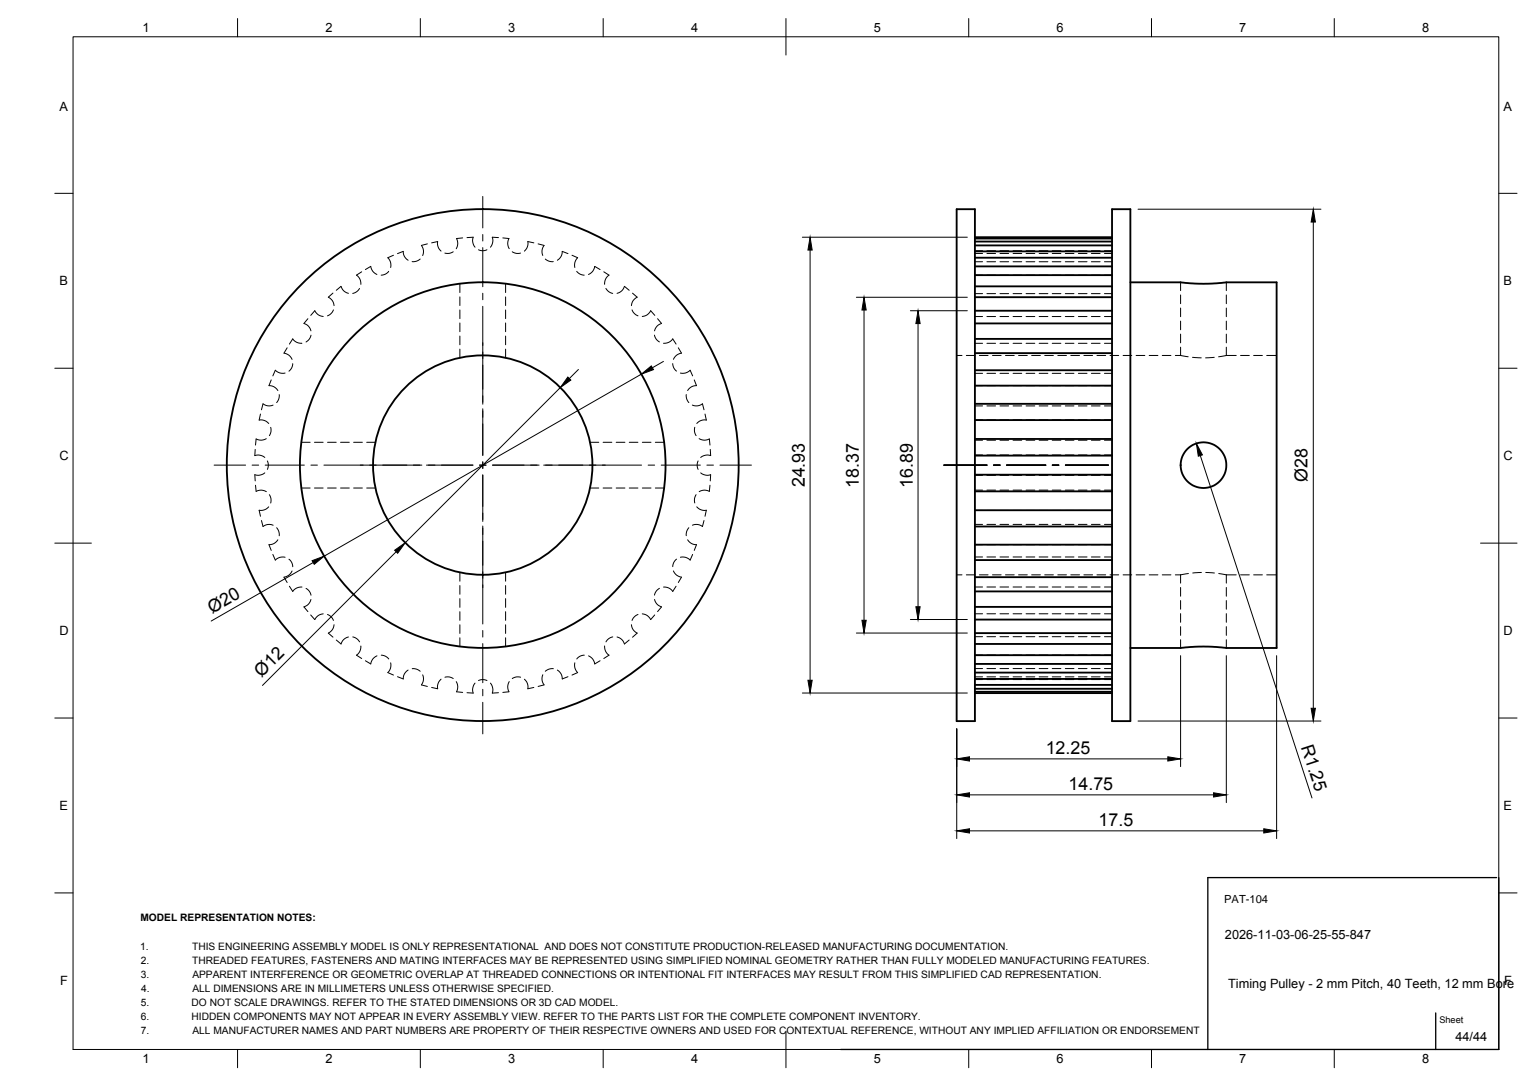
ISO-10303-21;
HEADER;
/* Generated by software containing ST-Developer
 * from STEP Tools, Inc. (www.steptools.com) 
 */

FILE_DESCRIPTION(
/* description */ ('Timing belt drive module 2 mm Pitch Timing 20T-40T'),

/* implementation_level */ '2;1');

FILE_NAME(
/* name */ 'Timing Pulley - 2 mm Pitch, 40 Teeth, 12 mm Bore.step',
/* time_stamp */ '2026-10-28T03:25:12-07:00',
/* author */ (''),
/* organization */ (''),
/* preprocessor_version */ 'ST-DEVELOPER v20.2',
/* originating_system */ 'Autodesk Translation Framework v15.17.0.0',
/* authorisation */ '');

FILE_SCHEMA (('AUTOMOTIVE_DESIGN { 1 0 10303 214 3 1 1 }'));
ENDSEC;

DATA;
#10=MECHANICAL_DESIGN_GEOMETRIC_PRESENTATION_REPRESENTATION('',(#580),#17830);
#363=B_SPLINE_CURVE_WITH_KNOTS('',3,(#16760,#16761,#16762,#16763,#16764,
#16765,#16766,#16767,#16768,#16769),.UNSPECIFIED.,.F.,.F.,(4,2,2,2,4),(0.565665723963061,
0.61280433739166,0.659942950820258,0.70708195805217,0.754220965284082),
 .UNSPECIFIED.);
#364=B_SPLINE_CURVE_WITH_KNOTS('',3,(#16771,#16772,#16773,#16774,#16775,
#16776,#16777,#16778,#16779,#16780,#16781,#16782,#16783,#16784,#16785,#16786,
#16787,#16788),.UNSPECIFIED.,.F.,.F.,(4,2,2,2,2,2,2,2,4),(0.18855524132102,
0.235693854749619,0.282832468178217,0.329971475410129,0.377110482642041,
0.424249489873953,0.471388497105864,0.518527110534463,0.565665723963061),
 .UNSPECIFIED.);
#365=B_SPLINE_CURVE_WITH_KNOTS('',3,(#16789,#16790,#16791,#16792,#16793,
#16794,#16795,#16796,#16797,#16798),.UNSPECIFIED.,.F.,.F.,(4,2,2,2,4),(0.754220965284082,
0.801359972515993,0.848498979747905,0.895637593176504,0.942776206605102),
 .UNSPECIFIED.);
#366=B_SPLINE_CURVE_WITH_KNOTS('',3,(#16802,#16803,#16804,#16805,#16806,
#16807,#16808,#16809,#16810,#16811),.UNSPECIFIED.,.F.,.F.,(4,2,2,2,4),(0.188940047579712,
0.236173496177583,0.283406944775455,0.330643519967439,0.377880095159423),
 .UNSPECIFIED.);
#367=B_SPLINE_CURVE_WITH_KNOTS('',3,(#16813,#16814,#16815,#16816,#16817,
#16818,#16819,#16820,#16821,#16822),.UNSPECIFIED.,.F.,.F.,(4,2,2,2,4),(0.,
0.0472365751919841,0.0944731503839682,0.14170659898184,0.188940047579712),
 .UNSPECIFIED.);
#368=B_SPLINE_CURVE_WITH_KNOTS('',3,(#16824,#16825,#16826,#16827,#16828,
#16829,#16830,#16831,#16832,#16833),.UNSPECIFIED.,.F.,.F.,(4,2,2,2,4),(0.566820142739135,
0.614053591337007,0.661287039934879,0.708523615126863,0.755760190318847),
 .UNSPECIFIED.);
#369=B_SPLINE_CURVE_WITH_KNOTS('',3,(#16834,#16835,#16836,#16837,#16838,
#16839,#16840,#16841,#16842,#16843),.UNSPECIFIED.,.F.,.F.,(4,2,2,2,4),(0.377880095159423,
0.425116670351408,0.472353245543392,0.519586694141263,0.566820142739135),
 .UNSPECIFIED.);
#370=B_SPLINE_CURVE_WITH_KNOTS('',3,(#16847,#16848,#16849,#16850,#16851,
#16852,#16853,#16854,#16855,#16856,#16857,#16858,#16859,#16860,#16861,#16862,
#16863,#16864),.UNSPECIFIED.,.F.,.F.,(4,2,2,2,2,2,2,2,4),(0.,0.0472365751919841,
0.0944731503839683,0.14170659898184,0.188940047579712,0.236173496177583,
0.283406944775455,0.330643519967439,0.377880095159423),.UNSPECIFIED.);
#371=B_SPLINE_CURVE_WITH_KNOTS('',3,(#16865,#16866,#16867,#16868,#16869,
#16870,#16871,#16872,#16873,#16874,#16875,#16876,#16877,#16878,#16879,#16880,
#16881,#16882),.UNSPECIFIED.,.F.,.F.,(4,2,2,2,2,2,2,2,4),(0.377880095159423,
0.425116670351408,0.472353245543392,0.519586694141263,0.566820142739135,
0.614053591337007,0.661287039934879,0.708523615126863,0.755760190318847),
 .UNSPECIFIED.);
#372=B_SPLINE_CURVE_WITH_KNOTS('',3,(#16886,#16887,#16888,#16889,#16890,
#16891,#16892,#16893,#16894,#16895),.UNSPECIFIED.,.F.,.F.,(4,2,2,2,4),(0.565665723963061,
0.61280433739166,0.659942950820258,0.70708195805217,0.754220965284082),
 .UNSPECIFIED.);
#373=B_SPLINE_CURVE_WITH_KNOTS('',3,(#16897,#16898,#16899,#16900,#16901,
#16902,#16903,#16904,#16905,#16906,#16907,#16908,#16909,#16910,#16911,#16912,
#16913,#16914),.UNSPECIFIED.,.F.,.F.,(4,2,2,2,2,2,2,2,4),(0.18855524132102,
0.235693854749619,0.282832468178217,0.329971475410129,0.377110482642041,
0.424249489873953,0.471388497105864,0.518527110534463,0.565665723963061),
 .UNSPECIFIED.);
#374=B_SPLINE_CURVE_WITH_KNOTS('',3,(#16915,#16916,#16917,#16918,#16919,
#16920,#16921,#16922,#16923,#16924),.UNSPECIFIED.,.F.,.F.,(4,2,2,2,4),(0.754220965284082,
0.801359972515993,0.848498979747905,0.895637593176504,0.942776206605102),
 .UNSPECIFIED.);
#375=B_SPLINE_CURVE_WITH_KNOTS('',3,(#16934,#16935,#16936,#16937,#16938,
#16939,#16940,#16941,#16942,#16943,#16944,#16945,#16946,#16947,#16948,#16949,
#16950,#16951),.UNSPECIFIED.,.F.,.F.,(4,2,2,2,2,2,2,2,4),(0.18855524132102,
0.235693854749619,0.282832468178217,0.329971475410129,0.377110482642041,
0.424249489873953,0.471388497105864,0.518527110534463,0.565665723963061),
 .UNSPECIFIED.);
#376=B_SPLINE_CURVE_WITH_KNOTS('',3,(#16953,#16954,#16955,#16956,#16957,
#16958,#16959,#16960,#16961,#16962),.UNSPECIFIED.,.F.,.F.,(4,2,2,2,4),(0.565665723963061,
0.61280433739166,0.659942950820258,0.70708195805217,0.754220965284082),
 .UNSPECIFIED.);
#377=B_SPLINE_CURVE_WITH_KNOTS('',3,(#16963,#16964,#16965,#16966,#16967,
#16968,#16969,#16970,#16971,#16972),.UNSPECIFIED.,.F.,.F.,(4,2,2,2,4),(0.754220965284082,
0.801359972515993,0.848498979747905,0.895637593176504,0.942776206605102),
 .UNSPECIFIED.);
#378=B_SPLINE_CURVE_WITH_KNOTS('',3,(#16975,#16976,#16977,#16978,#16979,
#16980,#16981,#16982,#16983,#16984,#16985,#16986,#16987,#16988,#16989,#16990,
#16991,#16992),.UNSPECIFIED.,.F.,.F.,(4,2,2,2,2,2,2,2,4),(0.18855524132102,
0.235693854749619,0.282832468178217,0.329971475410129,0.377110482642041,
0.424249489873953,0.471388497105864,0.518527110534463,0.565665723963061),
 .UNSPECIFIED.);
#379=B_SPLINE_CURVE_WITH_KNOTS('',3,(#16994,#16995,#16996,#16997,#16998,
#16999,#17000,#17001,#17002,#17003),.UNSPECIFIED.,.F.,.F.,(4,2,2,2,4),(0.565665723963061,
0.61280433739166,0.659942950820258,0.70708195805217,0.754220965284082),
 .UNSPECIFIED.);
#380=B_SPLINE_CURVE_WITH_KNOTS('',3,(#17004,#17005,#17006,#17007,#17008,
#17009,#17010,#17011,#17012,#17013),.UNSPECIFIED.,.F.,.F.,(4,2,2,2,4),(0.754220965284082,
0.801359972515993,0.848498979747905,0.895637593176504,0.942776206605102),
 .UNSPECIFIED.);
#381=B_SPLINE_CURVE_WITH_KNOTS('',3,(#17018,#17019,#17020,#17021,#17022,
#17023,#17024,#17025,#17026,#17027,#17028,#17029,#17030,#17031,#17032,#17033,
#17034,#17035),.UNSPECIFIED.,.F.,.F.,(4,2,2,2,2,2,2,2,4),(0.,0.0472365751919841,
0.0944731503839683,0.14170659898184,0.188940047579712,0.236173496177583,
0.283406944775455,0.330643519967439,0.377880095159424),.UNSPECIFIED.);
#382=B_SPLINE_CURVE_WITH_KNOTS('',3,(#17036,#17037,#17038,#17039,#17040,
#17041,#17042,#17043,#17044,#17045,#17046,#17047,#17048,#17049,#17050,#17051,
#17052,#17053),.UNSPECIFIED.,.F.,.F.,(4,2,2,2,2,2,2,2,4),(0.377880095159424,
0.425116670351408,0.472353245543392,0.519586694141263,0.566820142739135,
0.614053591337007,0.661287039934879,0.708523615126863,0.755760190318847),
 .UNSPECIFIED.);
#383=B_SPLINE_CURVE_WITH_KNOTS('',3,(#17057,#17058,#17059,#17060,#17061,
#17062,#17063,#17064,#17065,#17066,#17067,#17068,#17069,#17070,#17071,#17072,
#17073,#17074),.UNSPECIFIED.,.F.,.F.,(4,2,2,2,2,2,2,2,4),(0.,0.0472365751919841,
0.0944731503839683,0.14170659898184,0.188940047579712,0.236173496177583,
0.283406944775455,0.330643519967439,0.377880095159423),.UNSPECIFIED.);
#384=B_SPLINE_CURVE_WITH_KNOTS('',3,(#17075,#17076,#17077,#17078,#17079,
#17080,#17081,#17082,#17083,#17084,#17085,#17086,#17087,#17088,#17089,#17090,
#17091,#17092),.UNSPECIFIED.,.F.,.F.,(4,2,2,2,2,2,2,2,4),(0.377880095159423,
0.425116670351408,0.472353245543392,0.519586694141263,0.566820142739135,
0.614053591337007,0.661287039934879,0.708523615126863,0.755760190318847),
 .UNSPECIFIED.);
#479=SHAPE_REPRESENTATION_RELATIONSHIP('SRR','None',#18053,#522);
#522=ADVANCED_BREP_SHAPE_REPRESENTATION('',(#636),#17828);
#580=STYLED_ITEM('',(#18310),#636);
#636=MANIFOLD_SOLID_BREP('Body1',#9039);
#761=FACE_BOUND('',#2021,.T.);
#762=FACE_BOUND('',#2022,.T.);
#763=FACE_BOUND('',#2023,.T.);
#764=FACE_BOUND('',#2027,.T.);
#765=FACE_BOUND('',#2028,.T.);
#766=FACE_BOUND('',#2029,.T.);
#767=FACE_BOUND('',#2031,.T.);
#768=FACE_BOUND('',#2033,.T.);
#769=FACE_BOUND('',#2036,.T.);
#770=FACE_BOUND('',#2038,.T.);
#771=FACE_BOUND('',#2041,.T.);
#946=PLANE('',#10469);
#947=PLANE('',#10470);
#948=PLANE('',#10554);
#949=PLANE('',#10555);
#950=PLANE('',#10639);
#1373=FACE_OUTER_BOUND('',#2018,.T.);
#1374=FACE_OUTER_BOUND('',#2019,.T.);
#1375=FACE_OUTER_BOUND('',#2020,.T.);
#1376=FACE_OUTER_BOUND('',#2024,.T.);
#1377=FACE_OUTER_BOUND('',#2025,.T.);
#1378=FACE_OUTER_BOUND('',#2026,.T.);
#1379=FACE_OUTER_BOUND('',#2030,.T.);
#1380=FACE_OUTER_BOUND('',#2032,.T.);
#1381=FACE_OUTER_BOUND('',#2034,.T.);
#1382=FACE_OUTER_BOUND('',#2035,.T.);
#1383=FACE_OUTER_BOUND('',#2037,.T.);
#1384=FACE_OUTER_BOUND('',#2039,.T.);
#1385=FACE_OUTER_BOUND('',#2040,.T.);
#1386=FACE_OUTER_BOUND('',#2042,.T.);
#1387=FACE_OUTER_BOUND('',#2043,.T.);
#1388=FACE_OUTER_BOUND('',#2044,.T.);
#1389=FACE_OUTER_BOUND('',#2045,.T.);
#1390=FACE_OUTER_BOUND('',#2046,.T.);
#1391=FACE_OUTER_BOUND('',#2047,.T.);
#1392=FACE_OUTER_BOUND('',#2048,.T.);
#1393=FACE_OUTER_BOUND('',#2049,.T.);
#1394=FACE_OUTER_BOUND('',#2050,.T.);
#1395=FACE_OUTER_BOUND('',#2051,.T.);
#1396=FACE_OUTER_BOUND('',#2052,.T.);
#1397=FACE_OUTER_BOUND('',#2053,.T.);
#1398=FACE_OUTER_BOUND('',#2054,.T.);
#1399=FACE_OUTER_BOUND('',#2055,.T.);
#1400=FACE_OUTER_BOUND('',#2056,.T.);
#1401=FACE_OUTER_BOUND('',#2057,.T.);
#1402=FACE_OUTER_BOUND('',#2058,.T.);
#1403=FACE_OUTER_BOUND('',#2059,.T.);
#1404=FACE_OUTER_BOUND('',#2060,.T.);
#1405=FACE_OUTER_BOUND('',#2061,.T.);
#1406=FACE_OUTER_BOUND('',#2062,.T.);
#1407=FACE_OUTER_BOUND('',#2063,.T.);
#1408=FACE_OUTER_BOUND('',#2064,.T.);
#1409=FACE_OUTER_BOUND('',#2065,.T.);
#1410=FACE_OUTER_BOUND('',#2066,.T.);
#1411=FACE_OUTER_BOUND('',#2067,.T.);
#1412=FACE_OUTER_BOUND('',#2068,.T.);
#1413=FACE_OUTER_BOUND('',#2069,.T.);
#1414=FACE_OUTER_BOUND('',#2070,.T.);
#1415=FACE_OUTER_BOUND('',#2071,.T.);
#1416=FACE_OUTER_BOUND('',#2072,.T.);
#1417=FACE_OUTER_BOUND('',#2073,.T.);
#1418=FACE_OUTER_BOUND('',#2074,.T.);
#1419=FACE_OUTER_BOUND('',#2075,.T.);
#1420=FACE_OUTER_BOUND('',#2076,.T.);
#1421=FACE_OUTER_BOUND('',#2077,.T.);
#1422=FACE_OUTER_BOUND('',#2078,.T.);
#1423=FACE_OUTER_BOUND('',#2079,.T.);
#1424=FACE_OUTER_BOUND('',#2080,.T.);
#1425=FACE_OUTER_BOUND('',#2081,.T.);
#1426=FACE_OUTER_BOUND('',#2082,.T.);
#1427=FACE_OUTER_BOUND('',#2083,.T.);
#1428=FACE_OUTER_BOUND('',#2084,.T.);
#1429=FACE_OUTER_BOUND('',#2085,.T.);
#1430=FACE_OUTER_BOUND('',#2086,.T.);
#1431=FACE_OUTER_BOUND('',#2087,.T.);
#1432=FACE_OUTER_BOUND('',#2088,.T.);
#1433=FACE_OUTER_BOUND('',#2089,.T.);
#1434=FACE_OUTER_BOUND('',#2090,.T.);
#1435=FACE_OUTER_BOUND('',#2091,.T.);
#1436=FACE_OUTER_BOUND('',#2092,.T.);
#1437=FACE_OUTER_BOUND('',#2093,.T.);
#1438=FACE_OUTER_BOUND('',#2094,.T.);
#1439=FACE_OUTER_BOUND('',#2095,.T.);
#1440=FACE_OUTER_BOUND('',#2096,.T.);
#1441=FACE_OUTER_BOUND('',#2097,.T.);
#1442=FACE_OUTER_BOUND('',#2098,.T.);
#1443=FACE_OUTER_BOUND('',#2099,.T.);
#1444=FACE_OUTER_BOUND('',#2100,.T.);
#1445=FACE_OUTER_BOUND('',#2101,.T.);
#1446=FACE_OUTER_BOUND('',#2102,.T.);
#1447=FACE_OUTER_BOUND('',#2103,.T.);
#1448=FACE_OUTER_BOUND('',#2104,.T.);
#1449=FACE_OUTER_BOUND('',#2105,.T.);
#1450=FACE_OUTER_BOUND('',#2106,.T.);
#1451=FACE_OUTER_BOUND('',#2107,.T.);
#1452=FACE_OUTER_BOUND('',#2108,.T.);
#1453=FACE_OUTER_BOUND('',#2109,.T.);
#1454=FACE_OUTER_BOUND('',#2110,.T.);
#1455=FACE_OUTER_BOUND('',#2111,.T.);
#1456=FACE_OUTER_BOUND('',#2112,.T.);
#1457=FACE_OUTER_BOUND('',#2113,.T.);
#1458=FACE_OUTER_BOUND('',#2114,.T.);
#1459=FACE_OUTER_BOUND('',#2115,.T.);
#1460=FACE_OUTER_BOUND('',#2116,.T.);
#1461=FACE_OUTER_BOUND('',#2117,.T.);
#1462=FACE_OUTER_BOUND('',#2118,.T.);
#1463=FACE_OUTER_BOUND('',#2119,.T.);
#1464=FACE_OUTER_BOUND('',#2120,.T.);
#1465=FACE_OUTER_BOUND('',#2121,.T.);
#2018=EDGE_LOOP('',(#7557,#7558,#7559,#7560,#7561,#7562,#7563,#7564,#7565));
#2019=EDGE_LOOP('',(#7566,#7567,#7568,#7569,#7570,#7571,#7572));
#2020=EDGE_LOOP('',(#7573,#7574,#7575,#7576,#7577,#7578,#7579,#7580,#7581));
#2021=EDGE_LOOP('',(#7582,#7583,#7584));
#2022=EDGE_LOOP('',(#7585,#7586,#7587));
#2023=EDGE_LOOP('',(#7588,#7589,#7590));
#2024=EDGE_LOOP('',(#7591,#7592,#7593,#7594,#7595,#7596,#7597));
#2025=EDGE_LOOP('',(#7598,#7599,#7600,#7601,#7602,#7603,#7604));
#2026=EDGE_LOOP('',(#7605,#7606,#7607,#7608,#7609,#7610,#7611,#7612,#7613,
#7614));
#2027=EDGE_LOOP('',(#7615,#7616));
#2028=EDGE_LOOP('',(#7617,#7618));
#2029=EDGE_LOOP('',(#7619,#7620));
#2030=EDGE_LOOP('',(#7621));
#2031=EDGE_LOOP('',(#7622));
#2032=EDGE_LOOP('',(#7623));
#2033=EDGE_LOOP('',(#7624,#7625,#7626,#7627,#7628,#7629,#7630,#7631,#7632,
#7633,#7634,#7635,#7636,#7637,#7638,#7639,#7640,#7641,#7642,#7643,#7644,
#7645,#7646,#7647,#7648,#7649,#7650,#7651,#7652,#7653,#7654,#7655,#7656,
#7657,#7658,#7659,#7660,#7661,#7662,#7663,#7664,#7665,#7666,#7667,#7668,
#7669,#7670,#7671,#7672,#7673,#7674,#7675,#7676,#7677,#7678,#7679,#7680,
#7681,#7682,#7683,#7684,#7685,#7686,#7687,#7688,#7689,#7690,#7691,#7692,
#7693,#7694,#7695,#7696,#7697,#7698,#7699,#7700,#7701,#7702,#7703));
#2034=EDGE_LOOP('',(#7704,#7705,#7706,#7707));
#2035=EDGE_LOOP('',(#7708));
#2036=EDGE_LOOP('',(#7709));
#2037=EDGE_LOOP('',(#7710));
#2038=EDGE_LOOP('',(#7711,#7712,#7713,#7714,#7715,#7716,#7717,#7718,#7719,
#7720,#7721,#7722,#7723,#7724,#7725,#7726,#7727,#7728,#7729,#7730,#7731,
#7732,#7733,#7734,#7735,#7736,#7737,#7738,#7739,#7740,#7741,#7742,#7743,
#7744,#7745,#7746,#7747,#7748,#7749,#7750,#7751,#7752,#7753,#7754,#7755,
#7756,#7757,#7758,#7759,#7760,#7761,#7762,#7763,#7764,#7765,#7766,#7767,
#7768,#7769,#7770,#7771,#7772,#7773,#7774,#7775,#7776,#7777,#7778,#7779,
#7780,#7781,#7782,#7783,#7784,#7785,#7786,#7787,#7788,#7789,#7790));
#2039=EDGE_LOOP('',(#7791,#7792,#7793,#7794));
#2040=EDGE_LOOP('',(#7795));
#2041=EDGE_LOOP('',(#7796));
#2042=EDGE_LOOP('',(#7797,#7798,#7799,#7800));
#2043=EDGE_LOOP('',(#7801,#7802,#7803,#7804));
#2044=EDGE_LOOP('',(#7805,#7806,#7807,#7808));
#2045=EDGE_LOOP('',(#7809,#7810,#7811,#7812));
#2046=EDGE_LOOP('',(#7813,#7814,#7815,#7816));
#2047=EDGE_LOOP('',(#7817,#7818,#7819,#7820));
#2048=EDGE_LOOP('',(#7821,#7822,#7823,#7824));
#2049=EDGE_LOOP('',(#7825,#7826,#7827,#7828));
#2050=EDGE_LOOP('',(#7829,#7830,#7831,#7832));
#2051=EDGE_LOOP('',(#7833,#7834,#7835,#7836));
#2052=EDGE_LOOP('',(#7837,#7838,#7839,#7840));
#2053=EDGE_LOOP('',(#7841,#7842,#7843,#7844));
#2054=EDGE_LOOP('',(#7845,#7846,#7847,#7848));
#2055=EDGE_LOOP('',(#7849,#7850,#7851,#7852));
#2056=EDGE_LOOP('',(#7853,#7854,#7855,#7856));
#2057=EDGE_LOOP('',(#7857,#7858,#7859,#7860));
#2058=EDGE_LOOP('',(#7861,#7862,#7863,#7864));
#2059=EDGE_LOOP('',(#7865,#7866,#7867,#7868));
#2060=EDGE_LOOP('',(#7869,#7870,#7871,#7872));
#2061=EDGE_LOOP('',(#7873,#7874,#7875,#7876));
#2062=EDGE_LOOP('',(#7877,#7878,#7879,#7880));
#2063=EDGE_LOOP('',(#7881,#7882,#7883,#7884));
#2064=EDGE_LOOP('',(#7885,#7886,#7887,#7888));
#2065=EDGE_LOOP('',(#7889,#7890,#7891,#7892));
#2066=EDGE_LOOP('',(#7893,#7894,#7895,#7896));
#2067=EDGE_LOOP('',(#7897,#7898,#7899,#7900));
#2068=EDGE_LOOP('',(#7901,#7902,#7903,#7904));
#2069=EDGE_LOOP('',(#7905,#7906,#7907,#7908));
#2070=EDGE_LOOP('',(#7909,#7910,#7911,#7912));
#2071=EDGE_LOOP('',(#7913,#7914,#7915,#7916));
#2072=EDGE_LOOP('',(#7917,#7918,#7919,#7920));
#2073=EDGE_LOOP('',(#7921,#7922,#7923,#7924));
#2074=EDGE_LOOP('',(#7925,#7926,#7927,#7928));
#2075=EDGE_LOOP('',(#7929,#7930,#7931,#7932));
#2076=EDGE_LOOP('',(#7933,#7934,#7935,#7936));
#2077=EDGE_LOOP('',(#7937,#7938,#7939,#7940));
#2078=EDGE_LOOP('',(#7941,#7942,#7943,#7944));
#2079=EDGE_LOOP('',(#7945,#7946,#7947,#7948));
#2080=EDGE_LOOP('',(#7949,#7950,#7951,#7952));
#2081=EDGE_LOOP('',(#7953,#7954,#7955,#7956));
#2082=EDGE_LOOP('',(#7957,#7958,#7959,#7960));
#2083=EDGE_LOOP('',(#7961,#7962,#7963,#7964));
#2084=EDGE_LOOP('',(#7965,#7966,#7967,#7968));
#2085=EDGE_LOOP('',(#7969,#7970,#7971,#7972));
#2086=EDGE_LOOP('',(#7973,#7974,#7975,#7976));
#2087=EDGE_LOOP('',(#7977,#7978,#7979,#7980));
#2088=EDGE_LOOP('',(#7981,#7982,#7983,#7984));
#2089=EDGE_LOOP('',(#7985,#7986,#7987,#7988));
#2090=EDGE_LOOP('',(#7989,#7990,#7991,#7992));
#2091=EDGE_LOOP('',(#7993,#7994,#7995,#7996));
#2092=EDGE_LOOP('',(#7997,#7998,#7999,#8000));
#2093=EDGE_LOOP('',(#8001,#8002,#8003,#8004));
#2094=EDGE_LOOP('',(#8005,#8006,#8007,#8008));
#2095=EDGE_LOOP('',(#8009,#8010,#8011,#8012));
#2096=EDGE_LOOP('',(#8013,#8014,#8015,#8016));
#2097=EDGE_LOOP('',(#8017,#8018,#8019,#8020));
#2098=EDGE_LOOP('',(#8021,#8022,#8023,#8024));
#2099=EDGE_LOOP('',(#8025,#8026,#8027,#8028));
#2100=EDGE_LOOP('',(#8029,#8030,#8031,#8032));
#2101=EDGE_LOOP('',(#8033,#8034,#8035,#8036));
#2102=EDGE_LOOP('',(#8037,#8038,#8039,#8040));
#2103=EDGE_LOOP('',(#8041,#8042,#8043,#8044));
#2104=EDGE_LOOP('',(#8045,#8046,#8047,#8048));
#2105=EDGE_LOOP('',(#8049,#8050,#8051,#8052));
#2106=EDGE_LOOP('',(#8053,#8054,#8055,#8056));
#2107=EDGE_LOOP('',(#8057,#8058,#8059,#8060));
#2108=EDGE_LOOP('',(#8061,#8062,#8063,#8064));
#2109=EDGE_LOOP('',(#8065,#8066,#8067,#8068));
#2110=EDGE_LOOP('',(#8069,#8070,#8071,#8072));
#2111=EDGE_LOOP('',(#8073,#8074,#8075,#8076));
#2112=EDGE_LOOP('',(#8077,#8078,#8079,#8080));
#2113=EDGE_LOOP('',(#8081,#8082,#8083,#8084));
#2114=EDGE_LOOP('',(#8085,#8086,#8087,#8088));
#2115=EDGE_LOOP('',(#8089,#8090,#8091,#8092));
#2116=EDGE_LOOP('',(#8093,#8094,#8095,#8096));
#2117=EDGE_LOOP('',(#8097,#8098,#8099,#8100));
#2118=EDGE_LOOP('',(#8101,#8102,#8103,#8104));
#2119=EDGE_LOOP('',(#8105,#8106,#8107,#8108));
#2120=EDGE_LOOP('',(#8109,#8110,#8111,#8112));
#2121=EDGE_LOOP('',(#8113,#8114,#8115,#8116));
#2614=CIRCLE('',#10462,1.);
#2615=CIRCLE('',#10463,1.);
#2616=CIRCLE('',#10467,0.6);
#2617=CIRCLE('',#10468,0.6);
#2618=CIRCLE('',#10471,1.4);
#2619=CIRCLE('',#10472,0.0555000000000001);
#2620=CIRCLE('',#10473,1.24783954473516);
#2621=CIRCLE('',#10474,0.0555000000000001);
#2622=CIRCLE('',#10475,1.24783954473516);
#2623=CIRCLE('',#10476,0.0555000000000001);
#2624=CIRCLE('',#10477,1.24783954473516);
#2625=CIRCLE('',#10478,0.0555000000000001);
#2626=CIRCLE('',#10479,1.24783954473516);
#2627=CIRCLE('',#10480,0.0555000000000001);
#2628=CIRCLE('',#10481,1.24783954473516);
#2629=CIRCLE('',#10482,0.0555000000000001);
#2630=CIRCLE('',#10483,1.24783954473516);
#2631=CIRCLE('',#10484,0.0555000000000001);
#2632=CIRCLE('',#10485,1.24783954473516);
#2633=CIRCLE('',#10486,0.0555000000000001);
#2634=CIRCLE('',#10487,1.24783954473516);
#2635=CIRCLE('',#10488,0.0555000000000001);
#2636=CIRCLE('',#10489,1.24783954473516);
#2637=CIRCLE('',#10490,0.0555000000000001);
#2638=CIRCLE('',#10491,1.24783954473516);
#2639=CIRCLE('',#10492,0.0555000000000001);
#2640=CIRCLE('',#10493,1.24783954473516);
#2641=CIRCLE('',#10494,0.0555000000000001);
#2642=CIRCLE('',#10495,1.24783954473516);
#2643=CIRCLE('',#10496,0.0555000000000001);
#2644=CIRCLE('',#10497,1.24783954473516);
#2645=CIRCLE('',#10498,0.0555000000000001);
#2646=CIRCLE('',#10499,1.24783954473516);
#2647=CIRCLE('',#10500,0.0555000000000001);
#2648=CIRCLE('',#10501,1.24783954473516);
#2649=CIRCLE('',#10502,0.0555000000000001);
#2650=CIRCLE('',#10503,1.24783954473516);
#2651=CIRCLE('',#10504,0.0555000000000001);
#2652=CIRCLE('',#10505,1.24783954473516);
#2653=CIRCLE('',#10506,0.0555000000000001);
#2654=CIRCLE('',#10507,1.24783954473516);
#2655=CIRCLE('',#10508,0.0555000000000001);
#2656=CIRCLE('',#10509,1.24783954473516);
#2657=CIRCLE('',#10510,0.0555000000000001);
#2658=CIRCLE('',#10511,1.24783954473516);
#2659=CIRCLE('',#10512,0.0555000000000001);
#2660=CIRCLE('',#10513,1.24783954473516);
#2661=CIRCLE('',#10514,0.0555000000000001);
#2662=CIRCLE('',#10515,1.24783954473516);
#2663=CIRCLE('',#10516,0.0555000000000001);
#2664=CIRCLE('',#10517,1.24783954473516);
#2665=CIRCLE('',#10518,0.0555000000000001);
#2666=CIRCLE('',#10519,1.24783954473516);
#2667=CIRCLE('',#10520,0.0555000000000001);
#2668=CIRCLE('',#10521,1.24783954473516);
#2669=CIRCLE('',#10522,0.0555000000000001);
#2670=CIRCLE('',#10523,1.24783954473516);
#2671=CIRCLE('',#10524,0.0555000000000001);
#2672=CIRCLE('',#10525,1.24783954473516);
#2673=CIRCLE('',#10526,0.0555000000000001);
#2674=CIRCLE('',#10527,1.24783954473516);
#2675=CIRCLE('',#10528,0.0555000000000001);
#2676=CIRCLE('',#10529,1.24783954473516);
#2677=CIRCLE('',#10530,0.0555000000000001);
#2678=CIRCLE('',#10531,1.24783954473516);
#2679=CIRCLE('',#10532,0.0555000000000001);
#2680=CIRCLE('',#10533,1.24783954473516);
#2681=CIRCLE('',#10534,0.0555000000000001);
#2682=CIRCLE('',#10535,1.24783954473516);
#2683=CIRCLE('',#10536,0.0555000000000001);
#2684=CIRCLE('',#10537,1.24783954473516);
#2685=CIRCLE('',#10538,0.0555000000000001);
#2686=CIRCLE('',#10539,1.24783954473516);
#2687=CIRCLE('',#10540,0.0555000000000001);
#2688=CIRCLE('',#10541,1.24783954473516);
#2689=CIRCLE('',#10542,0.0555000000000001);
#2690=CIRCLE('',#10543,1.24783954473516);
#2691=CIRCLE('',#10544,0.0555000000000001);
#2692=CIRCLE('',#10545,1.24783954473516);
#2693=CIRCLE('',#10546,0.0555000000000001);
#2694=CIRCLE('',#10547,1.24783954473516);
#2695=CIRCLE('',#10548,0.0555000000000001);
#2696=CIRCLE('',#10549,1.24783954473516);
#2697=CIRCLE('',#10550,0.0555000000000001);
#2698=CIRCLE('',#10551,1.24783954473516);
#2699=CIRCLE('',#10553,1.4);
#2700=CIRCLE('',#10556,1.4);
#2701=CIRCLE('',#10557,0.0555000000000001);
#2702=CIRCLE('',#10558,1.24783954473516);
#2703=CIRCLE('',#10559,0.0555000000000001);
#2704=CIRCLE('',#10560,1.24783954473516);
#2705=CIRCLE('',#10561,0.0555000000000001);
#2706=CIRCLE('',#10562,1.24783954473516);
#2707=CIRCLE('',#10563,0.0555000000000001);
#2708=CIRCLE('',#10564,1.24783954473516);
#2709=CIRCLE('',#10565,0.0555000000000001);
#2710=CIRCLE('',#10566,1.24783954473516);
#2711=CIRCLE('',#10567,0.0555000000000001);
#2712=CIRCLE('',#10568,1.24783954473516);
#2713=CIRCLE('',#10569,0.0555000000000001);
#2714=CIRCLE('',#10570,1.24783954473516);
#2715=CIRCLE('',#10571,0.0555000000000001);
#2716=CIRCLE('',#10572,1.24783954473516);
#2717=CIRCLE('',#10573,0.0555000000000001);
#2718=CIRCLE('',#10574,1.24783954473516);
#2719=CIRCLE('',#10575,0.0555000000000001);
#2720=CIRCLE('',#10576,1.24783954473516);
#2721=CIRCLE('',#10577,0.0555000000000001);
#2722=CIRCLE('',#10578,1.24783954473516);
#2723=CIRCLE('',#10579,0.0555000000000001);
#2724=CIRCLE('',#10580,1.24783954473516);
#2725=CIRCLE('',#10581,0.0555000000000001);
#2726=CIRCLE('',#10582,1.24783954473516);
#2727=CIRCLE('',#10583,0.0555000000000001);
#2728=CIRCLE('',#10584,1.24783954473516);
#2729=CIRCLE('',#10585,0.0555000000000001);
#2730=CIRCLE('',#10586,1.24783954473516);
#2731=CIRCLE('',#10587,0.0555000000000001);
#2732=CIRCLE('',#10588,1.24783954473516);
#2733=CIRCLE('',#10589,0.0555000000000001);
#2734=CIRCLE('',#10590,1.24783954473516);
#2735=CIRCLE('',#10591,0.0555000000000001);
#2736=CIRCLE('',#10592,1.24783954473516);
#2737=CIRCLE('',#10593,0.0555000000000001);
#2738=CIRCLE('',#10594,1.24783954473516);
#2739=CIRCLE('',#10595,0.0555000000000001);
#2740=CIRCLE('',#10596,1.24783954473516);
#2741=CIRCLE('',#10597,0.0555000000000001);
#2742=CIRCLE('',#10598,1.24783954473516);
#2743=CIRCLE('',#10599,0.0555000000000001);
#2744=CIRCLE('',#10600,1.24783954473516);
#2745=CIRCLE('',#10601,0.0555000000000001);
#2746=CIRCLE('',#10602,1.24783954473516);
#2747=CIRCLE('',#10603,0.0555000000000001);
#2748=CIRCLE('',#10604,1.24783954473516);
#2749=CIRCLE('',#10605,0.0555000000000001);
#2750=CIRCLE('',#10606,1.24783954473516);
#2751=CIRCLE('',#10607,0.0555000000000001);
#2752=CIRCLE('',#10608,1.24783954473516);
#2753=CIRCLE('',#10609,0.0555000000000001);
#2754=CIRCLE('',#10610,1.24783954473516);
#2755=CIRCLE('',#10611,0.0555000000000001);
#2756=CIRCLE('',#10612,1.24783954473516);
#2757=CIRCLE('',#10613,0.0555000000000001);
#2758=CIRCLE('',#10614,1.24783954473516);
#2759=CIRCLE('',#10615,0.0555000000000001);
#2760=CIRCLE('',#10616,1.24783954473516);
#2761=CIRCLE('',#10617,0.0555000000000001);
#2762=CIRCLE('',#10618,1.24783954473516);
#2763=CIRCLE('',#10619,0.0555000000000001);
#2764=CIRCLE('',#10620,1.24783954473516);
#2765=CIRCLE('',#10621,0.0555000000000001);
#2766=CIRCLE('',#10622,1.24783954473516);
#2767=CIRCLE('',#10623,0.0555000000000001);
#2768=CIRCLE('',#10624,1.24783954473516);
#2769=CIRCLE('',#10625,0.0555000000000001);
#2770=CIRCLE('',#10626,1.24783954473516);
#2771=CIRCLE('',#10627,0.0555000000000001);
#2772=CIRCLE('',#10628,1.24783954473516);
#2773=CIRCLE('',#10629,0.0555000000000001);
#2774=CIRCLE('',#10630,1.24783954473516);
#2775=CIRCLE('',#10631,0.0555000000000001);
#2776=CIRCLE('',#10632,1.24783954473516);
#2777=CIRCLE('',#10633,0.0555000000000001);
#2778=CIRCLE('',#10634,1.24783954473516);
#2779=CIRCLE('',#10635,0.0555000000000001);
#2780=CIRCLE('',#10636,1.24783954473516);
#2781=CIRCLE('',#10638,1.4);
#3154=LINE('',#16800,#3632);
#3155=LINE('',#16884,#3633);
#3156=LINE('',#16928,#3634);
#3157=LINE('',#16930,#3635);
#3158=LINE('',#17016,#3636);
#3159=LINE('',#17093,#3637);
#3160=LINE('',#17097,#3638);
#3161=LINE('',#17099,#3639);
#3162=LINE('',#17268,#3640);
#3163=LINE('',#17436,#3641);
#3164=LINE('',#17439,#3642);
#3165=LINE('',#17440,#3643);
#3166=LINE('',#17442,#3644);
#3167=LINE('',#17444,#3645);
#3168=LINE('',#17446,#3646);
#3169=LINE('',#17448,#3647);
#3170=LINE('',#17450,#3648);
#3171=LINE('',#17452,#3649);
#3172=LINE('',#17454,#3650);
#3173=LINE('',#17456,#3651);
#3174=LINE('',#17458,#3652);
#3175=LINE('',#17460,#3653);
#3176=LINE('',#17462,#3654);
#3177=LINE('',#17464,#3655);
#3178=LINE('',#17466,#3656);
#3179=LINE('',#17468,#3657);
#3180=LINE('',#17470,#3658);
#3181=LINE('',#17472,#3659);
#3182=LINE('',#17474,#3660);
#3183=LINE('',#17476,#3661);
#3184=LINE('',#17478,#3662);
#3185=LINE('',#17480,#3663);
#3186=LINE('',#17482,#3664);
#3187=LINE('',#17484,#3665);
#3188=LINE('',#17486,#3666);
#3189=LINE('',#17488,#3667);
#3190=LINE('',#17490,#3668);
#3191=LINE('',#17492,#3669);
#3192=LINE('',#17494,#3670);
#3193=LINE('',#17496,#3671);
#3194=LINE('',#17498,#3672);
#3195=LINE('',#17500,#3673);
#3196=LINE('',#17502,#3674);
#3197=LINE('',#17504,#3675);
#3198=LINE('',#17506,#3676);
#3199=LINE('',#17508,#3677);
#3200=LINE('',#17510,#3678);
#3201=LINE('',#17512,#3679);
#3202=LINE('',#17514,#3680);
#3203=LINE('',#17516,#3681);
#3204=LINE('',#17518,#3682);
#3205=LINE('',#17520,#3683);
#3206=LINE('',#17522,#3684);
#3207=LINE('',#17524,#3685);
#3208=LINE('',#17526,#3686);
#3209=LINE('',#17528,#3687);
#3210=LINE('',#17530,#3688);
#3211=LINE('',#17532,#3689);
#3212=LINE('',#17534,#3690);
#3213=LINE('',#17536,#3691);
#3214=LINE('',#17538,#3692);
#3215=LINE('',#17540,#3693);
#3216=LINE('',#17542,#3694);
#3217=LINE('',#17544,#3695);
#3218=LINE('',#17546,#3696);
#3219=LINE('',#17548,#3697);
#3220=LINE('',#17550,#3698);
#3221=LINE('',#17552,#3699);
#3222=LINE('',#17554,#3700);
#3223=LINE('',#17556,#3701);
#3224=LINE('',#17558,#3702);
#3225=LINE('',#17560,#3703);
#3226=LINE('',#17562,#3704);
#3227=LINE('',#17564,#3705);
#3228=LINE('',#17566,#3706);
#3229=LINE('',#17568,#3707);
#3230=LINE('',#17570,#3708);
#3231=LINE('',#17572,#3709);
#3232=LINE('',#17574,#3710);
#3233=LINE('',#17576,#3711);
#3234=LINE('',#17578,#3712);
#3235=LINE('',#17580,#3713);
#3236=LINE('',#17582,#3714);
#3237=LINE('',#17584,#3715);
#3238=LINE('',#17586,#3716);
#3239=LINE('',#17588,#3717);
#3240=LINE('',#17590,#3718);
#3241=LINE('',#17592,#3719);
#3242=LINE('',#17594,#3720);
#3243=LINE('',#17596,#3721);
#3632=VECTOR('',#13061,0.125);
#3633=VECTOR('',#13064,0.125);
#3634=VECTOR('',#13069,1.);
#3635=VECTOR('',#13070,1.);
#3636=VECTOR('',#13075,0.125);
#3637=VECTOR('',#13078,0.125);
#3638=VECTOR('',#13083,0.6);
#3639=VECTOR('',#13084,0.6);
#3640=VECTOR('',#13257,1.4);
#3641=VECTOR('',#13428,1.4);
#3642=VECTOR('',#13433,1.);
#3643=VECTOR('',#13434,1.);
#3644=VECTOR('',#13437,1.);
#3645=VECTOR('',#13440,1.);
#3646=VECTOR('',#13443,1.);
#3647=VECTOR('',#13446,1.);
#3648=VECTOR('',#13449,1.);
#3649=VECTOR('',#13452,1.);
#3650=VECTOR('',#13455,1.);
#3651=VECTOR('',#13458,1.);
#3652=VECTOR('',#13461,1.);
#3653=VECTOR('',#13464,1.);
#3654=VECTOR('',#13467,1.);
#3655=VECTOR('',#13470,1.);
#3656=VECTOR('',#13473,1.);
#3657=VECTOR('',#13476,1.);
#3658=VECTOR('',#13479,1.);
#3659=VECTOR('',#13482,1.);
#3660=VECTOR('',#13485,1.);
#3661=VECTOR('',#13488,1.);
#3662=VECTOR('',#13491,1.);
#3663=VECTOR('',#13494,1.);
#3664=VECTOR('',#13497,1.);
#3665=VECTOR('',#13500,1.);
#3666=VECTOR('',#13503,1.);
#3667=VECTOR('',#13506,1.);
#3668=VECTOR('',#13509,1.);
#3669=VECTOR('',#13512,1.);
#3670=VECTOR('',#13515,1.);
#3671=VECTOR('',#13518,1.);
#3672=VECTOR('',#13521,1.);
#3673=VECTOR('',#13524,1.);
#3674=VECTOR('',#13527,1.);
#3675=VECTOR('',#13530,1.);
#3676=VECTOR('',#13533,1.);
#3677=VECTOR('',#13536,1.);
#3678=VECTOR('',#13539,1.);
#3679=VECTOR('',#13542,1.);
#3680=VECTOR('',#13545,1.);
#3681=VECTOR('',#13548,1.);
#3682=VECTOR('',#13551,1.);
#3683=VECTOR('',#13554,1.);
#3684=VECTOR('',#13557,1.);
#3685=VECTOR('',#13560,1.);
#3686=VECTOR('',#13563,1.);
#3687=VECTOR('',#13566,1.);
#3688=VECTOR('',#13569,1.);
#3689=VECTOR('',#13572,1.);
#3690=VECTOR('',#13575,1.);
#3691=VECTOR('',#13578,1.);
#3692=VECTOR('',#13581,1.);
#3693=VECTOR('',#13584,1.);
#3694=VECTOR('',#13587,1.);
#3695=VECTOR('',#13590,1.);
#3696=VECTOR('',#13593,1.);
#3697=VECTOR('',#13596,1.);
#3698=VECTOR('',#13599,1.);
#3699=VECTOR('',#13602,1.);
#3700=VECTOR('',#13605,1.);
#3701=VECTOR('',#13608,1.);
#3702=VECTOR('',#13611,1.);
#3703=VECTOR('',#13614,1.);
#3704=VECTOR('',#13617,1.);
#3705=VECTOR('',#13620,1.);
#3706=VECTOR('',#13623,1.);
#3707=VECTOR('',#13626,1.);
#3708=VECTOR('',#13629,1.);
#3709=VECTOR('',#13632,1.);
#3710=VECTOR('',#13635,1.);
#3711=VECTOR('',#13638,1.);
#3712=VECTOR('',#13641,1.);
#3713=VECTOR('',#13644,1.);
#3714=VECTOR('',#13647,1.);
#3715=VECTOR('',#13650,1.);
#3716=VECTOR('',#13653,1.);
#3717=VECTOR('',#13656,1.);
#3718=VECTOR('',#13659,1.);
#3719=VECTOR('',#13662,1.);
#3720=VECTOR('',#13665,1.);
#3721=VECTOR('',#13668,1.);
#4359=VERTEX_POINT('',#16758);
#4360=VERTEX_POINT('',#16759);
#4361=VERTEX_POINT('',#16770);
#4362=VERTEX_POINT('',#16799);
#4363=VERTEX_POINT('',#16801);
#4364=VERTEX_POINT('',#16812);
#4365=VERTEX_POINT('',#16823);
#4366=VERTEX_POINT('',#16845);
#4367=VERTEX_POINT('',#16846);
#4368=VERTEX_POINT('',#16883);
#4369=VERTEX_POINT('',#16885);
#4370=VERTEX_POINT('',#16896);
#4371=VERTEX_POINT('',#16926);
#4372=VERTEX_POINT('',#16929);
#4373=VERTEX_POINT('',#16932);
#4374=VERTEX_POINT('',#16933);
#4375=VERTEX_POINT('',#16952);
#4376=VERTEX_POINT('',#16973);
#4377=VERTEX_POINT('',#16974);
#4378=VERTEX_POINT('',#16993);
#4379=VERTEX_POINT('',#17015);
#4380=VERTEX_POINT('',#17017);
#4381=VERTEX_POINT('',#17055);
#4382=VERTEX_POINT('',#17056);
#4383=VERTEX_POINT('',#17095);
#4384=VERTEX_POINT('',#17098);
#4385=VERTEX_POINT('',#17103);
#4386=VERTEX_POINT('',#17105);
#4387=VERTEX_POINT('',#17106);
#4388=VERTEX_POINT('',#17108);
#4389=VERTEX_POINT('',#17110);
#4390=VERTEX_POINT('',#17112);
#4391=VERTEX_POINT('',#17114);
#4392=VERTEX_POINT('',#17116);
#4393=VERTEX_POINT('',#17118);
#4394=VERTEX_POINT('',#17120);
#4395=VERTEX_POINT('',#17122);
#4396=VERTEX_POINT('',#17124);
#4397=VERTEX_POINT('',#17126);
#4398=VERTEX_POINT('',#17128);
#4399=VERTEX_POINT('',#17130);
#4400=VERTEX_POINT('',#17132);
#4401=VERTEX_POINT('',#17134);
#4402=VERTEX_POINT('',#17136);
#4403=VERTEX_POINT('',#17138);
#4404=VERTEX_POINT('',#17140);
#4405=VERTEX_POINT('',#17142);
#4406=VERTEX_POINT('',#17144);
#4407=VERTEX_POINT('',#17146);
#4408=VERTEX_POINT('',#17148);
#4409=VERTEX_POINT('',#17150);
#4410=VERTEX_POINT('',#17152);
#4411=VERTEX_POINT('',#17154);
#4412=VERTEX_POINT('',#17156);
#4413=VERTEX_POINT('',#17158);
#4414=VERTEX_POINT('',#17160);
#4415=VERTEX_POINT('',#17162);
#4416=VERTEX_POINT('',#17164);
#4417=VERTEX_POINT('',#17166);
#4418=VERTEX_POINT('',#17168);
#4419=VERTEX_POINT('',#17170);
#4420=VERTEX_POINT('',#17172);
#4421=VERTEX_POINT('',#17174);
#4422=VERTEX_POINT('',#17176);
#4423=VERTEX_POINT('',#17178);
#4424=VERTEX_POINT('',#17180);
#4425=VERTEX_POINT('',#17182);
#4426=VERTEX_POINT('',#17184);
#4427=VERTEX_POINT('',#17186);
#4428=VERTEX_POINT('',#17188);
#4429=VERTEX_POINT('',#17190);
#4430=VERTEX_POINT('',#17192);
#4431=VERTEX_POINT('',#17194);
#4432=VERTEX_POINT('',#17196);
#4433=VERTEX_POINT('',#17198);
#4434=VERTEX_POINT('',#17200);
#4435=VERTEX_POINT('',#17202);
#4436=VERTEX_POINT('',#17204);
#4437=VERTEX_POINT('',#17206);
#4438=VERTEX_POINT('',#17208);
#4439=VERTEX_POINT('',#17210);
#4440=VERTEX_POINT('',#17212);
#4441=VERTEX_POINT('',#17214);
#4442=VERTEX_POINT('',#17216);
#4443=VERTEX_POINT('',#17218);
#4444=VERTEX_POINT('',#17220);
#4445=VERTEX_POINT('',#17222);
#4446=VERTEX_POINT('',#17224);
#4447=VERTEX_POINT('',#17226);
#4448=VERTEX_POINT('',#17228);
#4449=VERTEX_POINT('',#17230);
#4450=VERTEX_POINT('',#17232);
#4451=VERTEX_POINT('',#17234);
#4452=VERTEX_POINT('',#17236);
#4453=VERTEX_POINT('',#17238);
#4454=VERTEX_POINT('',#17240);
#4455=VERTEX_POINT('',#17242);
#4456=VERTEX_POINT('',#17244);
#4457=VERTEX_POINT('',#17246);
#4458=VERTEX_POINT('',#17248);
#4459=VERTEX_POINT('',#17250);
#4460=VERTEX_POINT('',#17252);
#4461=VERTEX_POINT('',#17254);
#4462=VERTEX_POINT('',#17256);
#4463=VERTEX_POINT('',#17258);
#4464=VERTEX_POINT('',#17260);
#4465=VERTEX_POINT('',#17262);
#4466=VERTEX_POINT('',#17266);
#4467=VERTEX_POINT('',#17271);
#4468=VERTEX_POINT('',#17273);
#4469=VERTEX_POINT('',#17274);
#4470=VERTEX_POINT('',#17276);
#4471=VERTEX_POINT('',#17278);
#4472=VERTEX_POINT('',#17280);
#4473=VERTEX_POINT('',#17282);
#4474=VERTEX_POINT('',#17284);
#4475=VERTEX_POINT('',#17286);
#4476=VERTEX_POINT('',#17288);
#4477=VERTEX_POINT('',#17290);
#4478=VERTEX_POINT('',#17292);
#4479=VERTEX_POINT('',#17294);
#4480=VERTEX_POINT('',#17296);
#4481=VERTEX_POINT('',#17298);
#4482=VERTEX_POINT('',#17300);
#4483=VERTEX_POINT('',#17302);
#4484=VERTEX_POINT('',#17304);
#4485=VERTEX_POINT('',#17306);
#4486=VERTEX_POINT('',#17308);
#4487=VERTEX_POINT('',#17310);
#4488=VERTEX_POINT('',#17312);
#4489=VERTEX_POINT('',#17314);
#4490=VERTEX_POINT('',#17316);
#4491=VERTEX_POINT('',#17318);
#4492=VERTEX_POINT('',#17320);
#4493=VERTEX_POINT('',#17322);
#4494=VERTEX_POINT('',#17324);
#4495=VERTEX_POINT('',#17326);
#4496=VERTEX_POINT('',#17328);
#4497=VERTEX_POINT('',#17330);
#4498=VERTEX_POINT('',#17332);
#4499=VERTEX_POINT('',#17334);
#4500=VERTEX_POINT('',#17336);
#4501=VERTEX_POINT('',#17338);
#4502=VERTEX_POINT('',#17340);
#4503=VERTEX_POINT('',#17342);
#4504=VERTEX_POINT('',#17344);
#4505=VERTEX_POINT('',#17346);
#4506=VERTEX_POINT('',#17348);
#4507=VERTEX_POINT('',#17350);
#4508=VERTEX_POINT('',#17352);
#4509=VERTEX_POINT('',#17354);
#4510=VERTEX_POINT('',#17356);
#4511=VERTEX_POINT('',#17358);
#4512=VERTEX_POINT('',#17360);
#4513=VERTEX_POINT('',#17362);
#4514=VERTEX_POINT('',#17364);
#4515=VERTEX_POINT('',#17366);
#4516=VERTEX_POINT('',#17368);
#4517=VERTEX_POINT('',#17370);
#4518=VERTEX_POINT('',#17372);
#4519=VERTEX_POINT('',#17374);
#4520=VERTEX_POINT('',#17376);
#4521=VERTEX_POINT('',#17378);
#4522=VERTEX_POINT('',#17380);
#4523=VERTEX_POINT('',#17382);
#4524=VERTEX_POINT('',#17384);
#4525=VERTEX_POINT('',#17386);
#4526=VERTEX_POINT('',#17388);
#4527=VERTEX_POINT('',#17390);
#4528=VERTEX_POINT('',#17392);
#4529=VERTEX_POINT('',#17394);
#4530=VERTEX_POINT('',#17396);
#4531=VERTEX_POINT('',#17398);
#4532=VERTEX_POINT('',#17400);
#4533=VERTEX_POINT('',#17402);
#4534=VERTEX_POINT('',#17404);
#4535=VERTEX_POINT('',#17406);
#4536=VERTEX_POINT('',#17408);
#4537=VERTEX_POINT('',#17410);
#4538=VERTEX_POINT('',#17412);
#4539=VERTEX_POINT('',#17414);
#4540=VERTEX_POINT('',#17416);
#4541=VERTEX_POINT('',#17418);
#4542=VERTEX_POINT('',#17420);
#4543=VERTEX_POINT('',#17422);
#4544=VERTEX_POINT('',#17424);
#4545=VERTEX_POINT('',#17426);
#4546=VERTEX_POINT('',#17428);
#4547=VERTEX_POINT('',#17430);
#4548=VERTEX_POINT('',#17434);
#5461=EDGE_CURVE('',#4359,#4360,#363,.T.);
#5462=EDGE_CURVE('',#4361,#4359,#364,.T.);
#5463=EDGE_CURVE('',#4360,#4361,#365,.T.);
#5464=EDGE_CURVE('',#4360,#4362,#3154,.T.);
#5465=EDGE_CURVE('',#4363,#4362,#366,.T.);
#5466=EDGE_CURVE('',#4364,#4363,#367,.T.);
#5467=EDGE_CURVE('',#4365,#4364,#368,.T.);
#5468=EDGE_CURVE('',#4362,#4365,#369,.T.);
#5469=EDGE_CURVE('',#4366,#4367,#370,.T.);
#5470=EDGE_CURVE('',#4367,#4366,#371,.T.);
#5471=EDGE_CURVE('',#4367,#4368,#3155,.T.);
#5472=EDGE_CURVE('',#4369,#4368,#372,.T.);
#5473=EDGE_CURVE('',#4370,#4369,#373,.T.);
#5474=EDGE_CURVE('',#4368,#4370,#374,.T.);
#5475=EDGE_CURVE('',#4371,#4371,#2614,.T.);
#5476=EDGE_CURVE('',#4371,#4361,#3156,.T.);
#5477=EDGE_CURVE('',#4359,#4372,#3157,.T.);
#5478=EDGE_CURVE('',#4372,#4372,#2615,.T.);
#5479=EDGE_CURVE('',#4373,#4374,#375,.T.);
#5480=EDGE_CURVE('',#4374,#4375,#376,.T.);
#5481=EDGE_CURVE('',#4375,#4373,#377,.T.);
#5482=EDGE_CURVE('',#4376,#4377,#378,.T.);
#5483=EDGE_CURVE('',#4377,#4378,#379,.T.);
#5484=EDGE_CURVE('',#4378,#4376,#380,.T.);
#5485=EDGE_CURVE('',#4375,#4379,#3158,.T.);
#5486=EDGE_CURVE('',#4380,#4379,#381,.T.);
#5487=EDGE_CURVE('',#4379,#4380,#382,.T.);
#5488=EDGE_CURVE('',#4381,#4382,#383,.T.);
#5489=EDGE_CURVE('',#4382,#4381,#384,.T.);
#5490=EDGE_CURVE('',#4382,#4378,#3159,.T.);
#5491=EDGE_CURVE('',#4383,#4383,#2616,.T.);
#5492=EDGE_CURVE('',#4383,#4363,#3160,.T.);
#5493=EDGE_CURVE('',#4365,#4384,#3161,.T.);
#5494=EDGE_CURVE('',#4384,#4384,#2617,.T.);
#5495=EDGE_CURVE('',#4385,#4385,#2618,.T.);
#5496=EDGE_CURVE('',#4386,#4387,#2619,.T.);
#5497=EDGE_CURVE('',#4388,#4387,#2620,.T.);
#5498=EDGE_CURVE('',#4388,#4389,#2621,.T.);
#5499=EDGE_CURVE('',#4390,#4389,#2622,.T.);
#5500=EDGE_CURVE('',#4390,#4391,#2623,.T.);
#5501=EDGE_CURVE('',#4392,#4391,#2624,.T.);
#5502=EDGE_CURVE('',#4392,#4393,#2625,.T.);
#5503=EDGE_CURVE('',#4394,#4393,#2626,.T.);
#5504=EDGE_CURVE('',#4394,#4395,#2627,.T.);
#5505=EDGE_CURVE('',#4396,#4395,#2628,.T.);
#5506=EDGE_CURVE('',#4396,#4397,#2629,.T.);
#5507=EDGE_CURVE('',#4398,#4397,#2630,.T.);
#5508=EDGE_CURVE('',#4398,#4399,#2631,.T.);
#5509=EDGE_CURVE('',#4400,#4399,#2632,.T.);
#5510=EDGE_CURVE('',#4400,#4401,#2633,.T.);
#5511=EDGE_CURVE('',#4402,#4401,#2634,.T.);
#5512=EDGE_CURVE('',#4402,#4403,#2635,.T.);
#5513=EDGE_CURVE('',#4404,#4403,#2636,.T.);
#5514=EDGE_CURVE('',#4404,#4405,#2637,.T.);
#5515=EDGE_CURVE('',#4406,#4405,#2638,.T.);
#5516=EDGE_CURVE('',#4406,#4407,#2639,.T.);
#5517=EDGE_CURVE('',#4408,#4407,#2640,.T.);
#5518=EDGE_CURVE('',#4408,#4409,#2641,.T.);
#5519=EDGE_CURVE('',#4410,#4409,#2642,.T.);
#5520=EDGE_CURVE('',#4410,#4411,#2643,.T.);
#5521=EDGE_CURVE('',#4412,#4411,#2644,.T.);
#5522=EDGE_CURVE('',#4412,#4413,#2645,.T.);
#5523=EDGE_CURVE('',#4414,#4413,#2646,.T.);
#5524=EDGE_CURVE('',#4414,#4415,#2647,.T.);
#5525=EDGE_CURVE('',#4416,#4415,#2648,.T.);
#5526=EDGE_CURVE('',#4416,#4417,#2649,.T.);
#5527=EDGE_CURVE('',#4418,#4417,#2650,.T.);
#5528=EDGE_CURVE('',#4418,#4419,#2651,.T.);
#5529=EDGE_CURVE('',#4420,#4419,#2652,.T.);
#5530=EDGE_CURVE('',#4420,#4421,#2653,.T.);
#5531=EDGE_CURVE('',#4422,#4421,#2654,.T.);
#5532=EDGE_CURVE('',#4422,#4423,#2655,.T.);
#5533=EDGE_CURVE('',#4424,#4423,#2656,.T.);
#5534=EDGE_CURVE('',#4424,#4425,#2657,.T.);
#5535=EDGE_CURVE('',#4426,#4425,#2658,.T.);
#5536=EDGE_CURVE('',#4426,#4427,#2659,.T.);
#5537=EDGE_CURVE('',#4428,#4427,#2660,.T.);
#5538=EDGE_CURVE('',#4428,#4429,#2661,.T.);
#5539=EDGE_CURVE('',#4430,#4429,#2662,.T.);
#5540=EDGE_CURVE('',#4430,#4431,#2663,.T.);
#5541=EDGE_CURVE('',#4432,#4431,#2664,.T.);
#5542=EDGE_CURVE('',#4432,#4433,#2665,.T.);
#5543=EDGE_CURVE('',#4434,#4433,#2666,.T.);
#5544=EDGE_CURVE('',#4434,#4435,#2667,.T.);
#5545=EDGE_CURVE('',#4436,#4435,#2668,.T.);
#5546=EDGE_CURVE('',#4436,#4437,#2669,.T.);
#5547=EDGE_CURVE('',#4438,#4437,#2670,.T.);
#5548=EDGE_CURVE('',#4438,#4439,#2671,.T.);
#5549=EDGE_CURVE('',#4440,#4439,#2672,.T.);
#5550=EDGE_CURVE('',#4440,#4441,#2673,.T.);
#5551=EDGE_CURVE('',#4442,#4441,#2674,.T.);
#5552=EDGE_CURVE('',#4442,#4443,#2675,.T.);
#5553=EDGE_CURVE('',#4444,#4443,#2676,.T.);
#5554=EDGE_CURVE('',#4444,#4445,#2677,.T.);
#5555=EDGE_CURVE('',#4446,#4445,#2678,.T.);
#5556=EDGE_CURVE('',#4446,#4447,#2679,.T.);
#5557=EDGE_CURVE('',#4448,#4447,#2680,.T.);
#5558=EDGE_CURVE('',#4448,#4449,#2681,.T.);
#5559=EDGE_CURVE('',#4450,#4449,#2682,.T.);
#5560=EDGE_CURVE('',#4450,#4451,#2683,.T.);
#5561=EDGE_CURVE('',#4452,#4451,#2684,.T.);
#5562=EDGE_CURVE('',#4452,#4453,#2685,.T.);
#5563=EDGE_CURVE('',#4454,#4453,#2686,.T.);
#5564=EDGE_CURVE('',#4454,#4455,#2687,.T.);
#5565=EDGE_CURVE('',#4456,#4455,#2688,.T.);
#5566=EDGE_CURVE('',#4456,#4457,#2689,.T.);
#5567=EDGE_CURVE('',#4458,#4457,#2690,.T.);
#5568=EDGE_CURVE('',#4458,#4459,#2691,.T.);
#5569=EDGE_CURVE('',#4460,#4459,#2692,.T.);
#5570=EDGE_CURVE('',#4460,#4461,#2693,.T.);
#5571=EDGE_CURVE('',#4462,#4461,#2694,.T.);
#5572=EDGE_CURVE('',#4462,#4463,#2695,.T.);
#5573=EDGE_CURVE('',#4464,#4463,#2696,.T.);
#5574=EDGE_CURVE('',#4464,#4465,#2697,.T.);
#5575=EDGE_CURVE('',#4386,#4465,#2698,.T.);
#5576=EDGE_CURVE('',#4466,#4466,#2699,.T.);
#5577=EDGE_CURVE('',#4466,#4385,#3162,.T.);
#5578=EDGE_CURVE('',#4467,#4467,#2700,.T.);
#5579=EDGE_CURVE('',#4468,#4469,#2701,.T.);
#5580=EDGE_CURVE('',#4469,#4470,#2702,.T.);
#5581=EDGE_CURVE('',#4470,#4471,#2703,.T.);
#5582=EDGE_CURVE('',#4471,#4472,#2704,.T.);
#5583=EDGE_CURVE('',#4472,#4473,#2705,.T.);
#5584=EDGE_CURVE('',#4473,#4474,#2706,.T.);
#5585=EDGE_CURVE('',#4474,#4475,#2707,.T.);
#5586=EDGE_CURVE('',#4475,#4476,#2708,.T.);
#5587=EDGE_CURVE('',#4476,#4477,#2709,.T.);
#5588=EDGE_CURVE('',#4477,#4478,#2710,.T.);
#5589=EDGE_CURVE('',#4478,#4479,#2711,.T.);
#5590=EDGE_CURVE('',#4479,#4480,#2712,.T.);
#5591=EDGE_CURVE('',#4480,#4481,#2713,.T.);
#5592=EDGE_CURVE('',#4481,#4482,#2714,.T.);
#5593=EDGE_CURVE('',#4482,#4483,#2715,.T.);
#5594=EDGE_CURVE('',#4483,#4484,#2716,.T.);
#5595=EDGE_CURVE('',#4484,#4485,#2717,.T.);
#5596=EDGE_CURVE('',#4485,#4486,#2718,.T.);
#5597=EDGE_CURVE('',#4486,#4487,#2719,.T.);
#5598=EDGE_CURVE('',#4487,#4488,#2720,.T.);
#5599=EDGE_CURVE('',#4488,#4489,#2721,.T.);
#5600=EDGE_CURVE('',#4489,#4490,#2722,.T.);
#5601=EDGE_CURVE('',#4490,#4491,#2723,.T.);
#5602=EDGE_CURVE('',#4491,#4492,#2724,.T.);
#5603=EDGE_CURVE('',#4492,#4493,#2725,.T.);
#5604=EDGE_CURVE('',#4493,#4494,#2726,.T.);
#5605=EDGE_CURVE('',#4494,#4495,#2727,.T.);
#5606=EDGE_CURVE('',#4495,#4496,#2728,.T.);
#5607=EDGE_CURVE('',#4496,#4497,#2729,.T.);
#5608=EDGE_CURVE('',#4497,#4498,#2730,.T.);
#5609=EDGE_CURVE('',#4498,#4499,#2731,.T.);
#5610=EDGE_CURVE('',#4499,#4500,#2732,.T.);
#5611=EDGE_CURVE('',#4500,#4501,#2733,.T.);
#5612=EDGE_CURVE('',#4501,#4502,#2734,.T.);
#5613=EDGE_CURVE('',#4502,#4503,#2735,.T.);
#5614=EDGE_CURVE('',#4503,#4504,#2736,.T.);
#5615=EDGE_CURVE('',#4504,#4505,#2737,.T.);
#5616=EDGE_CURVE('',#4505,#4506,#2738,.T.);
#5617=EDGE_CURVE('',#4506,#4507,#2739,.T.);
#5618=EDGE_CURVE('',#4507,#4508,#2740,.T.);
#5619=EDGE_CURVE('',#4508,#4509,#2741,.T.);
#5620=EDGE_CURVE('',#4509,#4510,#2742,.T.);
#5621=EDGE_CURVE('',#4510,#4511,#2743,.T.);
#5622=EDGE_CURVE('',#4511,#4512,#2744,.T.);
#5623=EDGE_CURVE('',#4512,#4513,#2745,.T.);
#5624=EDGE_CURVE('',#4513,#4514,#2746,.T.);
#5625=EDGE_CURVE('',#4514,#4515,#2747,.T.);
#5626=EDGE_CURVE('',#4515,#4516,#2748,.T.);
#5627=EDGE_CURVE('',#4516,#4517,#2749,.T.);
#5628=EDGE_CURVE('',#4517,#4518,#2750,.T.);
#5629=EDGE_CURVE('',#4518,#4519,#2751,.T.);
#5630=EDGE_CURVE('',#4519,#4520,#2752,.T.);
#5631=EDGE_CURVE('',#4520,#4521,#2753,.T.);
#5632=EDGE_CURVE('',#4521,#4522,#2754,.T.);
#5633=EDGE_CURVE('',#4522,#4523,#2755,.T.);
#5634=EDGE_CURVE('',#4523,#4524,#2756,.T.);
#5635=EDGE_CURVE('',#4524,#4525,#2757,.T.);
#5636=EDGE_CURVE('',#4525,#4526,#2758,.T.);
#5637=EDGE_CURVE('',#4526,#4527,#2759,.T.);
#5638=EDGE_CURVE('',#4527,#4528,#2760,.T.);
#5639=EDGE_CURVE('',#4528,#4529,#2761,.T.);
#5640=EDGE_CURVE('',#4529,#4530,#2762,.T.);
#5641=EDGE_CURVE('',#4530,#4531,#2763,.T.);
#5642=EDGE_CURVE('',#4531,#4532,#2764,.T.);
#5643=EDGE_CURVE('',#4532,#4533,#2765,.T.);
#5644=EDGE_CURVE('',#4533,#4534,#2766,.T.);
#5645=EDGE_CURVE('',#4534,#4535,#2767,.T.);
#5646=EDGE_CURVE('',#4535,#4536,#2768,.T.);
#5647=EDGE_CURVE('',#4536,#4537,#2769,.T.);
#5648=EDGE_CURVE('',#4537,#4538,#2770,.T.);
#5649=EDGE_CURVE('',#4538,#4539,#2771,.T.);
#5650=EDGE_CURVE('',#4539,#4540,#2772,.T.);
#5651=EDGE_CURVE('',#4540,#4541,#2773,.T.);
#5652=EDGE_CURVE('',#4541,#4542,#2774,.T.);
#5653=EDGE_CURVE('',#4542,#4543,#2775,.T.);
#5654=EDGE_CURVE('',#4543,#4544,#2776,.T.);
#5655=EDGE_CURVE('',#4544,#4545,#2777,.T.);
#5656=EDGE_CURVE('',#4545,#4546,#2778,.T.);
#5657=EDGE_CURVE('',#4546,#4547,#2779,.T.);
#5658=EDGE_CURVE('',#4547,#4468,#2780,.T.);
#5659=EDGE_CURVE('',#4548,#4548,#2781,.T.);
#5660=EDGE_CURVE('',#4548,#4467,#3163,.T.);
#5661=EDGE_CURVE('',#4469,#4386,#3164,.T.);
#5662=EDGE_CURVE('',#4387,#4468,#3165,.T.);
#5663=EDGE_CURVE('',#4547,#4388,#3166,.T.);
#5664=EDGE_CURVE('',#4389,#4546,#3167,.T.);
#5665=EDGE_CURVE('',#4545,#4390,#3168,.T.);
#5666=EDGE_CURVE('',#4391,#4544,#3169,.T.);
#5667=EDGE_CURVE('',#4543,#4392,#3170,.T.);
#5668=EDGE_CURVE('',#4393,#4542,#3171,.T.);
#5669=EDGE_CURVE('',#4541,#4394,#3172,.T.);
#5670=EDGE_CURVE('',#4395,#4540,#3173,.T.);
#5671=EDGE_CURVE('',#4539,#4396,#3174,.T.);
#5672=EDGE_CURVE('',#4397,#4538,#3175,.T.);
#5673=EDGE_CURVE('',#4537,#4398,#3176,.T.);
#5674=EDGE_CURVE('',#4399,#4536,#3177,.T.);
#5675=EDGE_CURVE('',#4535,#4400,#3178,.T.);
#5676=EDGE_CURVE('',#4401,#4534,#3179,.T.);
#5677=EDGE_CURVE('',#4533,#4402,#3180,.T.);
#5678=EDGE_CURVE('',#4403,#4532,#3181,.T.);
#5679=EDGE_CURVE('',#4531,#4404,#3182,.T.);
#5680=EDGE_CURVE('',#4405,#4530,#3183,.T.);
#5681=EDGE_CURVE('',#4529,#4406,#3184,.T.);
#5682=EDGE_CURVE('',#4407,#4528,#3185,.T.);
#5683=EDGE_CURVE('',#4527,#4408,#3186,.T.);
#5684=EDGE_CURVE('',#4409,#4526,#3187,.T.);
#5685=EDGE_CURVE('',#4525,#4410,#3188,.T.);
#5686=EDGE_CURVE('',#4411,#4524,#3189,.T.);
#5687=EDGE_CURVE('',#4523,#4412,#3190,.T.);
#5688=EDGE_CURVE('',#4413,#4522,#3191,.T.);
#5689=EDGE_CURVE('',#4521,#4414,#3192,.T.);
#5690=EDGE_CURVE('',#4415,#4520,#3193,.T.);
#5691=EDGE_CURVE('',#4519,#4416,#3194,.T.);
#5692=EDGE_CURVE('',#4417,#4518,#3195,.T.);
#5693=EDGE_CURVE('',#4517,#4418,#3196,.T.);
#5694=EDGE_CURVE('',#4419,#4516,#3197,.T.);
#5695=EDGE_CURVE('',#4515,#4420,#3198,.T.);
#5696=EDGE_CURVE('',#4421,#4514,#3199,.T.);
#5697=EDGE_CURVE('',#4513,#4422,#3200,.T.);
#5698=EDGE_CURVE('',#4423,#4512,#3201,.T.);
#5699=EDGE_CURVE('',#4511,#4424,#3202,.T.);
#5700=EDGE_CURVE('',#4425,#4510,#3203,.T.);
#5701=EDGE_CURVE('',#4509,#4426,#3204,.T.);
#5702=EDGE_CURVE('',#4427,#4508,#3205,.T.);
#5703=EDGE_CURVE('',#4507,#4428,#3206,.T.);
#5704=EDGE_CURVE('',#4429,#4506,#3207,.T.);
#5705=EDGE_CURVE('',#4505,#4430,#3208,.T.);
#5706=EDGE_CURVE('',#4431,#4504,#3209,.T.);
#5707=EDGE_CURVE('',#4503,#4432,#3210,.T.);
#5708=EDGE_CURVE('',#4433,#4502,#3211,.T.);
#5709=EDGE_CURVE('',#4501,#4434,#3212,.T.);
#5710=EDGE_CURVE('',#4435,#4500,#3213,.T.);
#5711=EDGE_CURVE('',#4499,#4436,#3214,.T.);
#5712=EDGE_CURVE('',#4437,#4498,#3215,.T.);
#5713=EDGE_CURVE('',#4497,#4438,#3216,.T.);
#5714=EDGE_CURVE('',#4439,#4496,#3217,.T.);
#5715=EDGE_CURVE('',#4495,#4440,#3218,.T.);
#5716=EDGE_CURVE('',#4441,#4494,#3219,.T.);
#5717=EDGE_CURVE('',#4493,#4442,#3220,.T.);
#5718=EDGE_CURVE('',#4443,#4492,#3221,.T.);
#5719=EDGE_CURVE('',#4491,#4444,#3222,.T.);
#5720=EDGE_CURVE('',#4445,#4490,#3223,.T.);
#5721=EDGE_CURVE('',#4489,#4446,#3224,.T.);
#5722=EDGE_CURVE('',#4447,#4488,#3225,.T.);
#5723=EDGE_CURVE('',#4487,#4448,#3226,.T.);
#5724=EDGE_CURVE('',#4449,#4486,#3227,.T.);
#5725=EDGE_CURVE('',#4485,#4450,#3228,.T.);
#5726=EDGE_CURVE('',#4451,#4484,#3229,.T.);
#5727=EDGE_CURVE('',#4483,#4452,#3230,.T.);
#5728=EDGE_CURVE('',#4453,#4482,#3231,.T.);
#5729=EDGE_CURVE('',#4481,#4454,#3232,.T.);
#5730=EDGE_CURVE('',#4455,#4480,#3233,.T.);
#5731=EDGE_CURVE('',#4479,#4456,#3234,.T.);
#5732=EDGE_CURVE('',#4457,#4478,#3235,.T.);
#5733=EDGE_CURVE('',#4477,#4458,#3236,.T.);
#5734=EDGE_CURVE('',#4459,#4476,#3237,.T.);
#5735=EDGE_CURVE('',#4475,#4460,#3238,.T.);
#5736=EDGE_CURVE('',#4461,#4474,#3239,.T.);
#5737=EDGE_CURVE('',#4473,#4462,#3240,.T.);
#5738=EDGE_CURVE('',#4463,#4472,#3241,.T.);
#5739=EDGE_CURVE('',#4465,#4470,#3242,.T.);
#5740=EDGE_CURVE('',#4471,#4464,#3243,.T.);
#7557=ORIENTED_EDGE('',*,*,#5461,.F.);
#7558=ORIENTED_EDGE('',*,*,#5462,.F.);
#7559=ORIENTED_EDGE('',*,*,#5463,.F.);
#7560=ORIENTED_EDGE('',*,*,#5464,.T.);
#7561=ORIENTED_EDGE('',*,*,#5465,.F.);
#7562=ORIENTED_EDGE('',*,*,#5466,.F.);
#7563=ORIENTED_EDGE('',*,*,#5467,.F.);
#7564=ORIENTED_EDGE('',*,*,#5468,.F.);
#7565=ORIENTED_EDGE('',*,*,#5464,.F.);
#7566=ORIENTED_EDGE('',*,*,#5469,.F.);
#7567=ORIENTED_EDGE('',*,*,#5470,.F.);
#7568=ORIENTED_EDGE('',*,*,#5471,.T.);
#7569=ORIENTED_EDGE('',*,*,#5472,.F.);
#7570=ORIENTED_EDGE('',*,*,#5473,.F.);
#7571=ORIENTED_EDGE('',*,*,#5474,.F.);
#7572=ORIENTED_EDGE('',*,*,#5471,.F.);
#7573=ORIENTED_EDGE('',*,*,#5475,.F.);
#7574=ORIENTED_EDGE('',*,*,#5476,.T.);
#7575=ORIENTED_EDGE('',*,*,#5462,.T.);
#7576=ORIENTED_EDGE('',*,*,#5477,.T.);
#7577=ORIENTED_EDGE('',*,*,#5478,.F.);
#7578=ORIENTED_EDGE('',*,*,#5477,.F.);
#7579=ORIENTED_EDGE('',*,*,#5461,.T.);
#7580=ORIENTED_EDGE('',*,*,#5463,.T.);
#7581=ORIENTED_EDGE('',*,*,#5476,.F.);
#7582=ORIENTED_EDGE('',*,*,#5473,.T.);
#7583=ORIENTED_EDGE('',*,*,#5472,.T.);
#7584=ORIENTED_EDGE('',*,*,#5474,.T.);
#7585=ORIENTED_EDGE('',*,*,#5479,.T.);
#7586=ORIENTED_EDGE('',*,*,#5480,.T.);
#7587=ORIENTED_EDGE('',*,*,#5481,.T.);
#7588=ORIENTED_EDGE('',*,*,#5482,.T.);
#7589=ORIENTED_EDGE('',*,*,#5483,.T.);
#7590=ORIENTED_EDGE('',*,*,#5484,.T.);
#7591=ORIENTED_EDGE('',*,*,#5480,.F.);
#7592=ORIENTED_EDGE('',*,*,#5479,.F.);
#7593=ORIENTED_EDGE('',*,*,#5481,.F.);
#7594=ORIENTED_EDGE('',*,*,#5485,.T.);
#7595=ORIENTED_EDGE('',*,*,#5486,.F.);
#7596=ORIENTED_EDGE('',*,*,#5487,.F.);
#7597=ORIENTED_EDGE('',*,*,#5485,.F.);
#7598=ORIENTED_EDGE('',*,*,#5488,.F.);
#7599=ORIENTED_EDGE('',*,*,#5489,.F.);
#7600=ORIENTED_EDGE('',*,*,#5490,.T.);
#7601=ORIENTED_EDGE('',*,*,#5483,.F.);
#7602=ORIENTED_EDGE('',*,*,#5482,.F.);
#7603=ORIENTED_EDGE('',*,*,#5484,.F.);
#7604=ORIENTED_EDGE('',*,*,#5490,.F.);
#7605=ORIENTED_EDGE('',*,*,#5491,.F.);
#7606=ORIENTED_EDGE('',*,*,#5492,.T.);
#7607=ORIENTED_EDGE('',*,*,#5465,.T.);
#7608=ORIENTED_EDGE('',*,*,#5468,.T.);
#7609=ORIENTED_EDGE('',*,*,#5493,.T.);
#7610=ORIENTED_EDGE('',*,*,#5494,.F.);
#7611=ORIENTED_EDGE('',*,*,#5493,.F.);
#7612=ORIENTED_EDGE('',*,*,#5467,.T.);
#7613=ORIENTED_EDGE('',*,*,#5466,.T.);
#7614=ORIENTED_EDGE('',*,*,#5492,.F.);
#7615=ORIENTED_EDGE('',*,*,#5469,.T.);
#7616=ORIENTED_EDGE('',*,*,#5470,.T.);
#7617=ORIENTED_EDGE('',*,*,#5488,.T.);
#7618=ORIENTED_EDGE('',*,*,#5489,.T.);
#7619=ORIENTED_EDGE('',*,*,#5486,.T.);
#7620=ORIENTED_EDGE('',*,*,#5487,.T.);
#7621=ORIENTED_EDGE('',*,*,#5475,.T.);
#7622=ORIENTED_EDGE('',*,*,#5491,.T.);
#7623=ORIENTED_EDGE('',*,*,#5495,.T.);
#7624=ORIENTED_EDGE('',*,*,#5496,.T.);
#7625=ORIENTED_EDGE('',*,*,#5497,.F.);
#7626=ORIENTED_EDGE('',*,*,#5498,.T.);
#7627=ORIENTED_EDGE('',*,*,#5499,.F.);
#7628=ORIENTED_EDGE('',*,*,#5500,.T.);
#7629=ORIENTED_EDGE('',*,*,#5501,.F.);
#7630=ORIENTED_EDGE('',*,*,#5502,.T.);
#7631=ORIENTED_EDGE('',*,*,#5503,.F.);
#7632=ORIENTED_EDGE('',*,*,#5504,.T.);
#7633=ORIENTED_EDGE('',*,*,#5505,.F.);
#7634=ORIENTED_EDGE('',*,*,#5506,.T.);
#7635=ORIENTED_EDGE('',*,*,#5507,.F.);
#7636=ORIENTED_EDGE('',*,*,#5508,.T.);
#7637=ORIENTED_EDGE('',*,*,#5509,.F.);
#7638=ORIENTED_EDGE('',*,*,#5510,.T.);
#7639=ORIENTED_EDGE('',*,*,#5511,.F.);
#7640=ORIENTED_EDGE('',*,*,#5512,.T.);
#7641=ORIENTED_EDGE('',*,*,#5513,.F.);
#7642=ORIENTED_EDGE('',*,*,#5514,.T.);
#7643=ORIENTED_EDGE('',*,*,#5515,.F.);
#7644=ORIENTED_EDGE('',*,*,#5516,.T.);
#7645=ORIENTED_EDGE('',*,*,#5517,.F.);
#7646=ORIENTED_EDGE('',*,*,#5518,.T.);
#7647=ORIENTED_EDGE('',*,*,#5519,.F.);
#7648=ORIENTED_EDGE('',*,*,#5520,.T.);
#7649=ORIENTED_EDGE('',*,*,#5521,.F.);
#7650=ORIENTED_EDGE('',*,*,#5522,.T.);
#7651=ORIENTED_EDGE('',*,*,#5523,.F.);
#7652=ORIENTED_EDGE('',*,*,#5524,.T.);
#7653=ORIENTED_EDGE('',*,*,#5525,.F.);
#7654=ORIENTED_EDGE('',*,*,#5526,.T.);
#7655=ORIENTED_EDGE('',*,*,#5527,.F.);
#7656=ORIENTED_EDGE('',*,*,#5528,.T.);
#7657=ORIENTED_EDGE('',*,*,#5529,.F.);
#7658=ORIENTED_EDGE('',*,*,#5530,.T.);
#7659=ORIENTED_EDGE('',*,*,#5531,.F.);
#7660=ORIENTED_EDGE('',*,*,#5532,.T.);
#7661=ORIENTED_EDGE('',*,*,#5533,.F.);
#7662=ORIENTED_EDGE('',*,*,#5534,.T.);
#7663=ORIENTED_EDGE('',*,*,#5535,.F.);
#7664=ORIENTED_EDGE('',*,*,#5536,.T.);
#7665=ORIENTED_EDGE('',*,*,#5537,.F.);
#7666=ORIENTED_EDGE('',*,*,#5538,.T.);
#7667=ORIENTED_EDGE('',*,*,#5539,.F.);
#7668=ORIENTED_EDGE('',*,*,#5540,.T.);
#7669=ORIENTED_EDGE('',*,*,#5541,.F.);
#7670=ORIENTED_EDGE('',*,*,#5542,.T.);
#7671=ORIENTED_EDGE('',*,*,#5543,.F.);
#7672=ORIENTED_EDGE('',*,*,#5544,.T.);
#7673=ORIENTED_EDGE('',*,*,#5545,.F.);
#7674=ORIENTED_EDGE('',*,*,#5546,.T.);
#7675=ORIENTED_EDGE('',*,*,#5547,.F.);
#7676=ORIENTED_EDGE('',*,*,#5548,.T.);
#7677=ORIENTED_EDGE('',*,*,#5549,.F.);
#7678=ORIENTED_EDGE('',*,*,#5550,.T.);
#7679=ORIENTED_EDGE('',*,*,#5551,.F.);
#7680=ORIENTED_EDGE('',*,*,#5552,.T.);
#7681=ORIENTED_EDGE('',*,*,#5553,.F.);
#7682=ORIENTED_EDGE('',*,*,#5554,.T.);
#7683=ORIENTED_EDGE('',*,*,#5555,.F.);
#7684=ORIENTED_EDGE('',*,*,#5556,.T.);
#7685=ORIENTED_EDGE('',*,*,#5557,.F.);
#7686=ORIENTED_EDGE('',*,*,#5558,.T.);
#7687=ORIENTED_EDGE('',*,*,#5559,.F.);
#7688=ORIENTED_EDGE('',*,*,#5560,.T.);
#7689=ORIENTED_EDGE('',*,*,#5561,.F.);
#7690=ORIENTED_EDGE('',*,*,#5562,.T.);
#7691=ORIENTED_EDGE('',*,*,#5563,.F.);
#7692=ORIENTED_EDGE('',*,*,#5564,.T.);
#7693=ORIENTED_EDGE('',*,*,#5565,.F.);
#7694=ORIENTED_EDGE('',*,*,#5566,.T.);
#7695=ORIENTED_EDGE('',*,*,#5567,.F.);
#7696=ORIENTED_EDGE('',*,*,#5568,.T.);
#7697=ORIENTED_EDGE('',*,*,#5569,.F.);
#7698=ORIENTED_EDGE('',*,*,#5570,.T.);
#7699=ORIENTED_EDGE('',*,*,#5571,.F.);
#7700=ORIENTED_EDGE('',*,*,#5572,.T.);
#7701=ORIENTED_EDGE('',*,*,#5573,.F.);
#7702=ORIENTED_EDGE('',*,*,#5574,.T.);
#7703=ORIENTED_EDGE('',*,*,#5575,.F.);
#7704=ORIENTED_EDGE('',*,*,#5576,.F.);
#7705=ORIENTED_EDGE('',*,*,#5577,.T.);
#7706=ORIENTED_EDGE('',*,*,#5495,.F.);
#7707=ORIENTED_EDGE('',*,*,#5577,.F.);
#7708=ORIENTED_EDGE('',*,*,#5576,.T.);
#7709=ORIENTED_EDGE('',*,*,#5478,.T.);
#7710=ORIENTED_EDGE('',*,*,#5578,.F.);
#7711=ORIENTED_EDGE('',*,*,#5579,.T.);
#7712=ORIENTED_EDGE('',*,*,#5580,.T.);
#7713=ORIENTED_EDGE('',*,*,#5581,.T.);
#7714=ORIENTED_EDGE('',*,*,#5582,.T.);
#7715=ORIENTED_EDGE('',*,*,#5583,.T.);
#7716=ORIENTED_EDGE('',*,*,#5584,.T.);
#7717=ORIENTED_EDGE('',*,*,#5585,.T.);
#7718=ORIENTED_EDGE('',*,*,#5586,.T.);
#7719=ORIENTED_EDGE('',*,*,#5587,.T.);
#7720=ORIENTED_EDGE('',*,*,#5588,.T.);
#7721=ORIENTED_EDGE('',*,*,#5589,.T.);
#7722=ORIENTED_EDGE('',*,*,#5590,.T.);
#7723=ORIENTED_EDGE('',*,*,#5591,.T.);
#7724=ORIENTED_EDGE('',*,*,#5592,.T.);
#7725=ORIENTED_EDGE('',*,*,#5593,.T.);
#7726=ORIENTED_EDGE('',*,*,#5594,.T.);
#7727=ORIENTED_EDGE('',*,*,#5595,.T.);
#7728=ORIENTED_EDGE('',*,*,#5596,.T.);
#7729=ORIENTED_EDGE('',*,*,#5597,.T.);
#7730=ORIENTED_EDGE('',*,*,#5598,.T.);
#7731=ORIENTED_EDGE('',*,*,#5599,.T.);
#7732=ORIENTED_EDGE('',*,*,#5600,.T.);
#7733=ORIENTED_EDGE('',*,*,#5601,.T.);
#7734=ORIENTED_EDGE('',*,*,#5602,.T.);
#7735=ORIENTED_EDGE('',*,*,#5603,.T.);
#7736=ORIENTED_EDGE('',*,*,#5604,.T.);
#7737=ORIENTED_EDGE('',*,*,#5605,.T.);
#7738=ORIENTED_EDGE('',*,*,#5606,.T.);
#7739=ORIENTED_EDGE('',*,*,#5607,.T.);
#7740=ORIENTED_EDGE('',*,*,#5608,.T.);
#7741=ORIENTED_EDGE('',*,*,#5609,.T.);
#7742=ORIENTED_EDGE('',*,*,#5610,.T.);
#7743=ORIENTED_EDGE('',*,*,#5611,.T.);
#7744=ORIENTED_EDGE('',*,*,#5612,.T.);
#7745=ORIENTED_EDGE('',*,*,#5613,.T.);
#7746=ORIENTED_EDGE('',*,*,#5614,.T.);
#7747=ORIENTED_EDGE('',*,*,#5615,.T.);
#7748=ORIENTED_EDGE('',*,*,#5616,.T.);
#7749=ORIENTED_EDGE('',*,*,#5617,.T.);
#7750=ORIENTED_EDGE('',*,*,#5618,.T.);
#7751=ORIENTED_EDGE('',*,*,#5619,.T.);
#7752=ORIENTED_EDGE('',*,*,#5620,.T.);
#7753=ORIENTED_EDGE('',*,*,#5621,.T.);
#7754=ORIENTED_EDGE('',*,*,#5622,.T.);
#7755=ORIENTED_EDGE('',*,*,#5623,.T.);
#7756=ORIENTED_EDGE('',*,*,#5624,.T.);
#7757=ORIENTED_EDGE('',*,*,#5625,.T.);
#7758=ORIENTED_EDGE('',*,*,#5626,.T.);
#7759=ORIENTED_EDGE('',*,*,#5627,.T.);
#7760=ORIENTED_EDGE('',*,*,#5628,.T.);
#7761=ORIENTED_EDGE('',*,*,#5629,.T.);
#7762=ORIENTED_EDGE('',*,*,#5630,.T.);
#7763=ORIENTED_EDGE('',*,*,#5631,.T.);
#7764=ORIENTED_EDGE('',*,*,#5632,.T.);
#7765=ORIENTED_EDGE('',*,*,#5633,.T.);
#7766=ORIENTED_EDGE('',*,*,#5634,.T.);
#7767=ORIENTED_EDGE('',*,*,#5635,.T.);
#7768=ORIENTED_EDGE('',*,*,#5636,.T.);
#7769=ORIENTED_EDGE('',*,*,#5637,.T.);
#7770=ORIENTED_EDGE('',*,*,#5638,.T.);
#7771=ORIENTED_EDGE('',*,*,#5639,.T.);
#7772=ORIENTED_EDGE('',*,*,#5640,.T.);
#7773=ORIENTED_EDGE('',*,*,#5641,.T.);
#7774=ORIENTED_EDGE('',*,*,#5642,.T.);
#7775=ORIENTED_EDGE('',*,*,#5643,.T.);
#7776=ORIENTED_EDGE('',*,*,#5644,.T.);
#7777=ORIENTED_EDGE('',*,*,#5645,.T.);
#7778=ORIENTED_EDGE('',*,*,#5646,.T.);
#7779=ORIENTED_EDGE('',*,*,#5647,.T.);
#7780=ORIENTED_EDGE('',*,*,#5648,.T.);
#7781=ORIENTED_EDGE('',*,*,#5649,.T.);
#7782=ORIENTED_EDGE('',*,*,#5650,.T.);
#7783=ORIENTED_EDGE('',*,*,#5651,.T.);
#7784=ORIENTED_EDGE('',*,*,#5652,.T.);
#7785=ORIENTED_EDGE('',*,*,#5653,.T.);
#7786=ORIENTED_EDGE('',*,*,#5654,.T.);
#7787=ORIENTED_EDGE('',*,*,#5655,.T.);
#7788=ORIENTED_EDGE('',*,*,#5656,.T.);
#7789=ORIENTED_EDGE('',*,*,#5657,.T.);
#7790=ORIENTED_EDGE('',*,*,#5658,.T.);
#7791=ORIENTED_EDGE('',*,*,#5659,.F.);
#7792=ORIENTED_EDGE('',*,*,#5660,.T.);
#7793=ORIENTED_EDGE('',*,*,#5578,.T.);
#7794=ORIENTED_EDGE('',*,*,#5660,.F.);
#7795=ORIENTED_EDGE('',*,*,#5659,.T.);
#7796=ORIENTED_EDGE('',*,*,#5494,.T.);
#7797=ORIENTED_EDGE('',*,*,#5661,.F.);
#7798=ORIENTED_EDGE('',*,*,#5579,.F.);
#7799=ORIENTED_EDGE('',*,*,#5662,.F.);
#7800=ORIENTED_EDGE('',*,*,#5496,.F.);
#7801=ORIENTED_EDGE('',*,*,#5662,.T.);
#7802=ORIENTED_EDGE('',*,*,#5658,.F.);
#7803=ORIENTED_EDGE('',*,*,#5663,.T.);
#7804=ORIENTED_EDGE('',*,*,#5497,.T.);
#7805=ORIENTED_EDGE('',*,*,#5663,.F.);
#7806=ORIENTED_EDGE('',*,*,#5657,.F.);
#7807=ORIENTED_EDGE('',*,*,#5664,.F.);
#7808=ORIENTED_EDGE('',*,*,#5498,.F.);
#7809=ORIENTED_EDGE('',*,*,#5664,.T.);
#7810=ORIENTED_EDGE('',*,*,#5656,.F.);
#7811=ORIENTED_EDGE('',*,*,#5665,.T.);
#7812=ORIENTED_EDGE('',*,*,#5499,.T.);
#7813=ORIENTED_EDGE('',*,*,#5665,.F.);
#7814=ORIENTED_EDGE('',*,*,#5655,.F.);
#7815=ORIENTED_EDGE('',*,*,#5666,.F.);
#7816=ORIENTED_EDGE('',*,*,#5500,.F.);
#7817=ORIENTED_EDGE('',*,*,#5666,.T.);
#7818=ORIENTED_EDGE('',*,*,#5654,.F.);
#7819=ORIENTED_EDGE('',*,*,#5667,.T.);
#7820=ORIENTED_EDGE('',*,*,#5501,.T.);
#7821=ORIENTED_EDGE('',*,*,#5667,.F.);
#7822=ORIENTED_EDGE('',*,*,#5653,.F.);
#7823=ORIENTED_EDGE('',*,*,#5668,.F.);
#7824=ORIENTED_EDGE('',*,*,#5502,.F.);
#7825=ORIENTED_EDGE('',*,*,#5668,.T.);
#7826=ORIENTED_EDGE('',*,*,#5652,.F.);
#7827=ORIENTED_EDGE('',*,*,#5669,.T.);
#7828=ORIENTED_EDGE('',*,*,#5503,.T.);
#7829=ORIENTED_EDGE('',*,*,#5669,.F.);
#7830=ORIENTED_EDGE('',*,*,#5651,.F.);
#7831=ORIENTED_EDGE('',*,*,#5670,.F.);
#7832=ORIENTED_EDGE('',*,*,#5504,.F.);
#7833=ORIENTED_EDGE('',*,*,#5670,.T.);
#7834=ORIENTED_EDGE('',*,*,#5650,.F.);
#7835=ORIENTED_EDGE('',*,*,#5671,.T.);
#7836=ORIENTED_EDGE('',*,*,#5505,.T.);
#7837=ORIENTED_EDGE('',*,*,#5671,.F.);
#7838=ORIENTED_EDGE('',*,*,#5649,.F.);
#7839=ORIENTED_EDGE('',*,*,#5672,.F.);
#7840=ORIENTED_EDGE('',*,*,#5506,.F.);
#7841=ORIENTED_EDGE('',*,*,#5672,.T.);
#7842=ORIENTED_EDGE('',*,*,#5648,.F.);
#7843=ORIENTED_EDGE('',*,*,#5673,.T.);
#7844=ORIENTED_EDGE('',*,*,#5507,.T.);
#7845=ORIENTED_EDGE('',*,*,#5673,.F.);
#7846=ORIENTED_EDGE('',*,*,#5647,.F.);
#7847=ORIENTED_EDGE('',*,*,#5674,.F.);
#7848=ORIENTED_EDGE('',*,*,#5508,.F.);
#7849=ORIENTED_EDGE('',*,*,#5674,.T.);
#7850=ORIENTED_EDGE('',*,*,#5646,.F.);
#7851=ORIENTED_EDGE('',*,*,#5675,.T.);
#7852=ORIENTED_EDGE('',*,*,#5509,.T.);
#7853=ORIENTED_EDGE('',*,*,#5675,.F.);
#7854=ORIENTED_EDGE('',*,*,#5645,.F.);
#7855=ORIENTED_EDGE('',*,*,#5676,.F.);
#7856=ORIENTED_EDGE('',*,*,#5510,.F.);
#7857=ORIENTED_EDGE('',*,*,#5676,.T.);
#7858=ORIENTED_EDGE('',*,*,#5644,.F.);
#7859=ORIENTED_EDGE('',*,*,#5677,.T.);
#7860=ORIENTED_EDGE('',*,*,#5511,.T.);
#7861=ORIENTED_EDGE('',*,*,#5677,.F.);
#7862=ORIENTED_EDGE('',*,*,#5643,.F.);
#7863=ORIENTED_EDGE('',*,*,#5678,.F.);
#7864=ORIENTED_EDGE('',*,*,#5512,.F.);
#7865=ORIENTED_EDGE('',*,*,#5678,.T.);
#7866=ORIENTED_EDGE('',*,*,#5642,.F.);
#7867=ORIENTED_EDGE('',*,*,#5679,.T.);
#7868=ORIENTED_EDGE('',*,*,#5513,.T.);
#7869=ORIENTED_EDGE('',*,*,#5679,.F.);
#7870=ORIENTED_EDGE('',*,*,#5641,.F.);
#7871=ORIENTED_EDGE('',*,*,#5680,.F.);
#7872=ORIENTED_EDGE('',*,*,#5514,.F.);
#7873=ORIENTED_EDGE('',*,*,#5680,.T.);
#7874=ORIENTED_EDGE('',*,*,#5640,.F.);
#7875=ORIENTED_EDGE('',*,*,#5681,.T.);
#7876=ORIENTED_EDGE('',*,*,#5515,.T.);
#7877=ORIENTED_EDGE('',*,*,#5681,.F.);
#7878=ORIENTED_EDGE('',*,*,#5639,.F.);
#7879=ORIENTED_EDGE('',*,*,#5682,.F.);
#7880=ORIENTED_EDGE('',*,*,#5516,.F.);
#7881=ORIENTED_EDGE('',*,*,#5682,.T.);
#7882=ORIENTED_EDGE('',*,*,#5638,.F.);
#7883=ORIENTED_EDGE('',*,*,#5683,.T.);
#7884=ORIENTED_EDGE('',*,*,#5517,.T.);
#7885=ORIENTED_EDGE('',*,*,#5683,.F.);
#7886=ORIENTED_EDGE('',*,*,#5637,.F.);
#7887=ORIENTED_EDGE('',*,*,#5684,.F.);
#7888=ORIENTED_EDGE('',*,*,#5518,.F.);
#7889=ORIENTED_EDGE('',*,*,#5684,.T.);
#7890=ORIENTED_EDGE('',*,*,#5636,.F.);
#7891=ORIENTED_EDGE('',*,*,#5685,.T.);
#7892=ORIENTED_EDGE('',*,*,#5519,.T.);
#7893=ORIENTED_EDGE('',*,*,#5685,.F.);
#7894=ORIENTED_EDGE('',*,*,#5635,.F.);
#7895=ORIENTED_EDGE('',*,*,#5686,.F.);
#7896=ORIENTED_EDGE('',*,*,#5520,.F.);
#7897=ORIENTED_EDGE('',*,*,#5686,.T.);
#7898=ORIENTED_EDGE('',*,*,#5634,.F.);
#7899=ORIENTED_EDGE('',*,*,#5687,.T.);
#7900=ORIENTED_EDGE('',*,*,#5521,.T.);
#7901=ORIENTED_EDGE('',*,*,#5687,.F.);
#7902=ORIENTED_EDGE('',*,*,#5633,.F.);
#7903=ORIENTED_EDGE('',*,*,#5688,.F.);
#7904=ORIENTED_EDGE('',*,*,#5522,.F.);
#7905=ORIENTED_EDGE('',*,*,#5688,.T.);
#7906=ORIENTED_EDGE('',*,*,#5632,.F.);
#7907=ORIENTED_EDGE('',*,*,#5689,.T.);
#7908=ORIENTED_EDGE('',*,*,#5523,.T.);
#7909=ORIENTED_EDGE('',*,*,#5689,.F.);
#7910=ORIENTED_EDGE('',*,*,#5631,.F.);
#7911=ORIENTED_EDGE('',*,*,#5690,.F.);
#7912=ORIENTED_EDGE('',*,*,#5524,.F.);
#7913=ORIENTED_EDGE('',*,*,#5690,.T.);
#7914=ORIENTED_EDGE('',*,*,#5630,.F.);
#7915=ORIENTED_EDGE('',*,*,#5691,.T.);
#7916=ORIENTED_EDGE('',*,*,#5525,.T.);
#7917=ORIENTED_EDGE('',*,*,#5691,.F.);
#7918=ORIENTED_EDGE('',*,*,#5629,.F.);
#7919=ORIENTED_EDGE('',*,*,#5692,.F.);
#7920=ORIENTED_EDGE('',*,*,#5526,.F.);
#7921=ORIENTED_EDGE('',*,*,#5692,.T.);
#7922=ORIENTED_EDGE('',*,*,#5628,.F.);
#7923=ORIENTED_EDGE('',*,*,#5693,.T.);
#7924=ORIENTED_EDGE('',*,*,#5527,.T.);
#7925=ORIENTED_EDGE('',*,*,#5693,.F.);
#7926=ORIENTED_EDGE('',*,*,#5627,.F.);
#7927=ORIENTED_EDGE('',*,*,#5694,.F.);
#7928=ORIENTED_EDGE('',*,*,#5528,.F.);
#7929=ORIENTED_EDGE('',*,*,#5694,.T.);
#7930=ORIENTED_EDGE('',*,*,#5626,.F.);
#7931=ORIENTED_EDGE('',*,*,#5695,.T.);
#7932=ORIENTED_EDGE('',*,*,#5529,.T.);
#7933=ORIENTED_EDGE('',*,*,#5695,.F.);
#7934=ORIENTED_EDGE('',*,*,#5625,.F.);
#7935=ORIENTED_EDGE('',*,*,#5696,.F.);
#7936=ORIENTED_EDGE('',*,*,#5530,.F.);
#7937=ORIENTED_EDGE('',*,*,#5696,.T.);
#7938=ORIENTED_EDGE('',*,*,#5624,.F.);
#7939=ORIENTED_EDGE('',*,*,#5697,.T.);
#7940=ORIENTED_EDGE('',*,*,#5531,.T.);
#7941=ORIENTED_EDGE('',*,*,#5697,.F.);
#7942=ORIENTED_EDGE('',*,*,#5623,.F.);
#7943=ORIENTED_EDGE('',*,*,#5698,.F.);
#7944=ORIENTED_EDGE('',*,*,#5532,.F.);
#7945=ORIENTED_EDGE('',*,*,#5698,.T.);
#7946=ORIENTED_EDGE('',*,*,#5622,.F.);
#7947=ORIENTED_EDGE('',*,*,#5699,.T.);
#7948=ORIENTED_EDGE('',*,*,#5533,.T.);
#7949=ORIENTED_EDGE('',*,*,#5699,.F.);
#7950=ORIENTED_EDGE('',*,*,#5621,.F.);
#7951=ORIENTED_EDGE('',*,*,#5700,.F.);
#7952=ORIENTED_EDGE('',*,*,#5534,.F.);
#7953=ORIENTED_EDGE('',*,*,#5700,.T.);
#7954=ORIENTED_EDGE('',*,*,#5620,.F.);
#7955=ORIENTED_EDGE('',*,*,#5701,.T.);
#7956=ORIENTED_EDGE('',*,*,#5535,.T.);
#7957=ORIENTED_EDGE('',*,*,#5701,.F.);
#7958=ORIENTED_EDGE('',*,*,#5619,.F.);
#7959=ORIENTED_EDGE('',*,*,#5702,.F.);
#7960=ORIENTED_EDGE('',*,*,#5536,.F.);
#7961=ORIENTED_EDGE('',*,*,#5702,.T.);
#7962=ORIENTED_EDGE('',*,*,#5618,.F.);
#7963=ORIENTED_EDGE('',*,*,#5703,.T.);
#7964=ORIENTED_EDGE('',*,*,#5537,.T.);
#7965=ORIENTED_EDGE('',*,*,#5703,.F.);
#7966=ORIENTED_EDGE('',*,*,#5617,.F.);
#7967=ORIENTED_EDGE('',*,*,#5704,.F.);
#7968=ORIENTED_EDGE('',*,*,#5538,.F.);
#7969=ORIENTED_EDGE('',*,*,#5704,.T.);
#7970=ORIENTED_EDGE('',*,*,#5616,.F.);
#7971=ORIENTED_EDGE('',*,*,#5705,.T.);
#7972=ORIENTED_EDGE('',*,*,#5539,.T.);
#7973=ORIENTED_EDGE('',*,*,#5705,.F.);
#7974=ORIENTED_EDGE('',*,*,#5615,.F.);
#7975=ORIENTED_EDGE('',*,*,#5706,.F.);
#7976=ORIENTED_EDGE('',*,*,#5540,.F.);
#7977=ORIENTED_EDGE('',*,*,#5706,.T.);
#7978=ORIENTED_EDGE('',*,*,#5614,.F.);
#7979=ORIENTED_EDGE('',*,*,#5707,.T.);
#7980=ORIENTED_EDGE('',*,*,#5541,.T.);
#7981=ORIENTED_EDGE('',*,*,#5707,.F.);
#7982=ORIENTED_EDGE('',*,*,#5613,.F.);
#7983=ORIENTED_EDGE('',*,*,#5708,.F.);
#7984=ORIENTED_EDGE('',*,*,#5542,.F.);
#7985=ORIENTED_EDGE('',*,*,#5708,.T.);
#7986=ORIENTED_EDGE('',*,*,#5612,.F.);
#7987=ORIENTED_EDGE('',*,*,#5709,.T.);
#7988=ORIENTED_EDGE('',*,*,#5543,.T.);
#7989=ORIENTED_EDGE('',*,*,#5709,.F.);
#7990=ORIENTED_EDGE('',*,*,#5611,.F.);
#7991=ORIENTED_EDGE('',*,*,#5710,.F.);
#7992=ORIENTED_EDGE('',*,*,#5544,.F.);
#7993=ORIENTED_EDGE('',*,*,#5710,.T.);
#7994=ORIENTED_EDGE('',*,*,#5610,.F.);
#7995=ORIENTED_EDGE('',*,*,#5711,.T.);
#7996=ORIENTED_EDGE('',*,*,#5545,.T.);
#7997=ORIENTED_EDGE('',*,*,#5711,.F.);
#7998=ORIENTED_EDGE('',*,*,#5609,.F.);
#7999=ORIENTED_EDGE('',*,*,#5712,.F.);
#8000=ORIENTED_EDGE('',*,*,#5546,.F.);
#8001=ORIENTED_EDGE('',*,*,#5712,.T.);
#8002=ORIENTED_EDGE('',*,*,#5608,.F.);
#8003=ORIENTED_EDGE('',*,*,#5713,.T.);
#8004=ORIENTED_EDGE('',*,*,#5547,.T.);
#8005=ORIENTED_EDGE('',*,*,#5713,.F.);
#8006=ORIENTED_EDGE('',*,*,#5607,.F.);
#8007=ORIENTED_EDGE('',*,*,#5714,.F.);
#8008=ORIENTED_EDGE('',*,*,#5548,.F.);
#8009=ORIENTED_EDGE('',*,*,#5714,.T.);
#8010=ORIENTED_EDGE('',*,*,#5606,.F.);
#8011=ORIENTED_EDGE('',*,*,#5715,.T.);
#8012=ORIENTED_EDGE('',*,*,#5549,.T.);
#8013=ORIENTED_EDGE('',*,*,#5715,.F.);
#8014=ORIENTED_EDGE('',*,*,#5605,.F.);
#8015=ORIENTED_EDGE('',*,*,#5716,.F.);
#8016=ORIENTED_EDGE('',*,*,#5550,.F.);
#8017=ORIENTED_EDGE('',*,*,#5716,.T.);
#8018=ORIENTED_EDGE('',*,*,#5604,.F.);
#8019=ORIENTED_EDGE('',*,*,#5717,.T.);
#8020=ORIENTED_EDGE('',*,*,#5551,.T.);
#8021=ORIENTED_EDGE('',*,*,#5717,.F.);
#8022=ORIENTED_EDGE('',*,*,#5603,.F.);
#8023=ORIENTED_EDGE('',*,*,#5718,.F.);
#8024=ORIENTED_EDGE('',*,*,#5552,.F.);
#8025=ORIENTED_EDGE('',*,*,#5718,.T.);
#8026=ORIENTED_EDGE('',*,*,#5602,.F.);
#8027=ORIENTED_EDGE('',*,*,#5719,.T.);
#8028=ORIENTED_EDGE('',*,*,#5553,.T.);
#8029=ORIENTED_EDGE('',*,*,#5719,.F.);
#8030=ORIENTED_EDGE('',*,*,#5601,.F.);
#8031=ORIENTED_EDGE('',*,*,#5720,.F.);
#8032=ORIENTED_EDGE('',*,*,#5554,.F.);
#8033=ORIENTED_EDGE('',*,*,#5720,.T.);
#8034=ORIENTED_EDGE('',*,*,#5600,.F.);
#8035=ORIENTED_EDGE('',*,*,#5721,.T.);
#8036=ORIENTED_EDGE('',*,*,#5555,.T.);
#8037=ORIENTED_EDGE('',*,*,#5721,.F.);
#8038=ORIENTED_EDGE('',*,*,#5599,.F.);
#8039=ORIENTED_EDGE('',*,*,#5722,.F.);
#8040=ORIENTED_EDGE('',*,*,#5556,.F.);
#8041=ORIENTED_EDGE('',*,*,#5722,.T.);
#8042=ORIENTED_EDGE('',*,*,#5598,.F.);
#8043=ORIENTED_EDGE('',*,*,#5723,.T.);
#8044=ORIENTED_EDGE('',*,*,#5557,.T.);
#8045=ORIENTED_EDGE('',*,*,#5723,.F.);
#8046=ORIENTED_EDGE('',*,*,#5597,.F.);
#8047=ORIENTED_EDGE('',*,*,#5724,.F.);
#8048=ORIENTED_EDGE('',*,*,#5558,.F.);
#8049=ORIENTED_EDGE('',*,*,#5724,.T.);
#8050=ORIENTED_EDGE('',*,*,#5596,.F.);
#8051=ORIENTED_EDGE('',*,*,#5725,.T.);
#8052=ORIENTED_EDGE('',*,*,#5559,.T.);
#8053=ORIENTED_EDGE('',*,*,#5725,.F.);
#8054=ORIENTED_EDGE('',*,*,#5595,.F.);
#8055=ORIENTED_EDGE('',*,*,#5726,.F.);
#8056=ORIENTED_EDGE('',*,*,#5560,.F.);
#8057=ORIENTED_EDGE('',*,*,#5726,.T.);
#8058=ORIENTED_EDGE('',*,*,#5594,.F.);
#8059=ORIENTED_EDGE('',*,*,#5727,.T.);
#8060=ORIENTED_EDGE('',*,*,#5561,.T.);
#8061=ORIENTED_EDGE('',*,*,#5727,.F.);
#8062=ORIENTED_EDGE('',*,*,#5593,.F.);
#8063=ORIENTED_EDGE('',*,*,#5728,.F.);
#8064=ORIENTED_EDGE('',*,*,#5562,.F.);
#8065=ORIENTED_EDGE('',*,*,#5728,.T.);
#8066=ORIENTED_EDGE('',*,*,#5592,.F.);
#8067=ORIENTED_EDGE('',*,*,#5729,.T.);
#8068=ORIENTED_EDGE('',*,*,#5563,.T.);
#8069=ORIENTED_EDGE('',*,*,#5729,.F.);
#8070=ORIENTED_EDGE('',*,*,#5591,.F.);
#8071=ORIENTED_EDGE('',*,*,#5730,.F.);
#8072=ORIENTED_EDGE('',*,*,#5564,.F.);
#8073=ORIENTED_EDGE('',*,*,#5730,.T.);
#8074=ORIENTED_EDGE('',*,*,#5590,.F.);
#8075=ORIENTED_EDGE('',*,*,#5731,.T.);
#8076=ORIENTED_EDGE('',*,*,#5565,.T.);
#8077=ORIENTED_EDGE('',*,*,#5731,.F.);
#8078=ORIENTED_EDGE('',*,*,#5589,.F.);
#8079=ORIENTED_EDGE('',*,*,#5732,.F.);
#8080=ORIENTED_EDGE('',*,*,#5566,.F.);
#8081=ORIENTED_EDGE('',*,*,#5732,.T.);
#8082=ORIENTED_EDGE('',*,*,#5588,.F.);
#8083=ORIENTED_EDGE('',*,*,#5733,.T.);
#8084=ORIENTED_EDGE('',*,*,#5567,.T.);
#8085=ORIENTED_EDGE('',*,*,#5733,.F.);
#8086=ORIENTED_EDGE('',*,*,#5587,.F.);
#8087=ORIENTED_EDGE('',*,*,#5734,.F.);
#8088=ORIENTED_EDGE('',*,*,#5568,.F.);
#8089=ORIENTED_EDGE('',*,*,#5734,.T.);
#8090=ORIENTED_EDGE('',*,*,#5586,.F.);
#8091=ORIENTED_EDGE('',*,*,#5735,.T.);
#8092=ORIENTED_EDGE('',*,*,#5569,.T.);
#8093=ORIENTED_EDGE('',*,*,#5735,.F.);
#8094=ORIENTED_EDGE('',*,*,#5585,.F.);
#8095=ORIENTED_EDGE('',*,*,#5736,.F.);
#8096=ORIENTED_EDGE('',*,*,#5570,.F.);
#8097=ORIENTED_EDGE('',*,*,#5736,.T.);
#8098=ORIENTED_EDGE('',*,*,#5584,.F.);
#8099=ORIENTED_EDGE('',*,*,#5737,.T.);
#8100=ORIENTED_EDGE('',*,*,#5571,.T.);
#8101=ORIENTED_EDGE('',*,*,#5738,.F.);
#8102=ORIENTED_EDGE('',*,*,#5572,.F.);
#8103=ORIENTED_EDGE('',*,*,#5737,.F.);
#8104=ORIENTED_EDGE('',*,*,#5583,.F.);
#8105=ORIENTED_EDGE('',*,*,#5661,.T.);
#8106=ORIENTED_EDGE('',*,*,#5575,.T.);
#8107=ORIENTED_EDGE('',*,*,#5739,.T.);
#8108=ORIENTED_EDGE('',*,*,#5580,.F.);
#8109=ORIENTED_EDGE('',*,*,#5740,.F.);
#8110=ORIENTED_EDGE('',*,*,#5581,.F.);
#8111=ORIENTED_EDGE('',*,*,#5739,.F.);
#8112=ORIENTED_EDGE('',*,*,#5574,.F.);
#8113=ORIENTED_EDGE('',*,*,#5738,.T.);
#8114=ORIENTED_EDGE('',*,*,#5582,.F.);
#8115=ORIENTED_EDGE('',*,*,#5740,.T.);
#8116=ORIENTED_EDGE('',*,*,#5573,.T.);
#8370=CYLINDRICAL_SURFACE('',#10459,0.125);
#8371=CYLINDRICAL_SURFACE('',#10460,0.125);
#8372=CYLINDRICAL_SURFACE('',#10461,1.);
#8373=CYLINDRICAL_SURFACE('',#10464,0.125);
#8374=CYLINDRICAL_SURFACE('',#10465,0.125);
#8375=CYLINDRICAL_SURFACE('',#10466,0.6);
#8376=CYLINDRICAL_SURFACE('',#10552,1.4);
#8377=CYLINDRICAL_SURFACE('',#10637,1.4);
#8378=CYLINDRICAL_SURFACE('',#10640,0.0555000000000001);
#8379=CYLINDRICAL_SURFACE('',#10641,1.24783954473516);
#8380=CYLINDRICAL_SURFACE('',#10642,0.0555000000000001);
#8381=CYLINDRICAL_SURFACE('',#10643,1.24783954473516);
#8382=CYLINDRICAL_SURFACE('',#10644,0.0555000000000001);
#8383=CYLINDRICAL_SURFACE('',#10645,1.24783954473516);
#8384=CYLINDRICAL_SURFACE('',#10646,0.0555000000000001);
#8385=CYLINDRICAL_SURFACE('',#10647,1.24783954473516);
#8386=CYLINDRICAL_SURFACE('',#10648,0.0555000000000001);
#8387=CYLINDRICAL_SURFACE('',#10649,1.24783954473516);
#8388=CYLINDRICAL_SURFACE('',#10650,0.0555000000000001);
#8389=CYLINDRICAL_SURFACE('',#10651,1.24783954473516);
#8390=CYLINDRICAL_SURFACE('',#10652,0.0555000000000001);
#8391=CYLINDRICAL_SURFACE('',#10653,1.24783954473516);
#8392=CYLINDRICAL_SURFACE('',#10654,0.0555000000000001);
#8393=CYLINDRICAL_SURFACE('',#10655,1.24783954473516);
#8394=CYLINDRICAL_SURFACE('',#10656,0.0555000000000001);
#8395=CYLINDRICAL_SURFACE('',#10657,1.24783954473516);
#8396=CYLINDRICAL_SURFACE('',#10658,0.0555000000000001);
#8397=CYLINDRICAL_SURFACE('',#10659,1.24783954473516);
#8398=CYLINDRICAL_SURFACE('',#10660,0.0555000000000001);
#8399=CYLINDRICAL_SURFACE('',#10661,1.24783954473516);
#8400=CYLINDRICAL_SURFACE('',#10662,0.0555000000000001);
#8401=CYLINDRICAL_SURFACE('',#10663,1.24783954473516);
#8402=CYLINDRICAL_SURFACE('',#10664,0.0555000000000001);
#8403=CYLINDRICAL_SURFACE('',#10665,1.24783954473516);
#8404=CYLINDRICAL_SURFACE('',#10666,0.0555000000000001);
#8405=CYLINDRICAL_SURFACE('',#10667,1.24783954473516);
#8406=CYLINDRICAL_SURFACE('',#10668,0.0555000000000001);
#8407=CYLINDRICAL_SURFACE('',#10669,1.24783954473516);
#8408=CYLINDRICAL_SURFACE('',#10670,0.0555000000000001);
#8409=CYLINDRICAL_SURFACE('',#10671,1.24783954473516);
#8410=CYLINDRICAL_SURFACE('',#10672,0.0555000000000001);
#8411=CYLINDRICAL_SURFACE('',#10673,1.24783954473516);
#8412=CYLINDRICAL_SURFACE('',#10674,0.0555000000000001);
#8413=CYLINDRICAL_SURFACE('',#10675,1.24783954473516);
#8414=CYLINDRICAL_SURFACE('',#10676,0.0555000000000001);
#8415=CYLINDRICAL_SURFACE('',#10677,1.24783954473516);
#8416=CYLINDRICAL_SURFACE('',#10678,0.0555000000000001);
#8417=CYLINDRICAL_SURFACE('',#10679,1.24783954473516);
#8418=CYLINDRICAL_SURFACE('',#10680,0.0555000000000001);
#8419=CYLINDRICAL_SURFACE('',#10681,1.24783954473516);
#8420=CYLINDRICAL_SURFACE('',#10682,0.0555000000000001);
#8421=CYLINDRICAL_SURFACE('',#10683,1.24783954473516);
#8422=CYLINDRICAL_SURFACE('',#10684,0.0555000000000001);
#8423=CYLINDRICAL_SURFACE('',#10685,1.24783954473516);
#8424=CYLINDRICAL_SURFACE('',#10686,0.0555000000000001);
#8425=CYLINDRICAL_SURFACE('',#10687,1.24783954473516);
#8426=CYLINDRICAL_SURFACE('',#10688,0.0555000000000001);
#8427=CYLINDRICAL_SURFACE('',#10689,1.24783954473516);
#8428=CYLINDRICAL_SURFACE('',#10690,0.0555000000000001);
#8429=CYLINDRICAL_SURFACE('',#10691,1.24783954473516);
#8430=CYLINDRICAL_SURFACE('',#10692,0.0555000000000001);
#8431=CYLINDRICAL_SURFACE('',#10693,1.24783954473516);
#8432=CYLINDRICAL_SURFACE('',#10694,0.0555000000000001);
#8433=CYLINDRICAL_SURFACE('',#10695,1.24783954473516);
#8434=CYLINDRICAL_SURFACE('',#10696,0.0555000000000001);
#8435=CYLINDRICAL_SURFACE('',#10697,1.24783954473516);
#8436=CYLINDRICAL_SURFACE('',#10698,0.0555000000000001);
#8437=CYLINDRICAL_SURFACE('',#10699,1.24783954473516);
#8438=CYLINDRICAL_SURFACE('',#10700,0.0555000000000001);
#8439=CYLINDRICAL_SURFACE('',#10701,1.24783954473516);
#8440=CYLINDRICAL_SURFACE('',#10702,0.0555000000000001);
#8441=CYLINDRICAL_SURFACE('',#10703,1.24783954473516);
#8442=CYLINDRICAL_SURFACE('',#10704,0.0555000000000001);
#8443=CYLINDRICAL_SURFACE('',#10705,1.24783954473516);
#8444=CYLINDRICAL_SURFACE('',#10706,0.0555000000000001);
#8445=CYLINDRICAL_SURFACE('',#10707,1.24783954473516);
#8446=CYLINDRICAL_SURFACE('',#10708,0.0555000000000001);
#8447=CYLINDRICAL_SURFACE('',#10709,1.24783954473516);
#8448=CYLINDRICAL_SURFACE('',#10710,0.0555000000000001);
#8449=CYLINDRICAL_SURFACE('',#10711,1.24783954473516);
#8450=CYLINDRICAL_SURFACE('',#10712,0.0555000000000001);
#8451=CYLINDRICAL_SURFACE('',#10713,1.24783954473516);
#8452=CYLINDRICAL_SURFACE('',#10714,0.0555000000000001);
#8453=CYLINDRICAL_SURFACE('',#10715,1.24783954473516);
#8454=CYLINDRICAL_SURFACE('',#10716,0.0555000000000001);
#8455=CYLINDRICAL_SURFACE('',#10717,1.24783954473516);
#8456=CYLINDRICAL_SURFACE('',#10718,0.0555000000000001);
#8457=CYLINDRICAL_SURFACE('',#10719,1.24783954473516);
#8871=ADVANCED_FACE('',(#1373),#8370,.F.);
#8872=ADVANCED_FACE('',(#1374),#8371,.F.);
#8873=ADVANCED_FACE('',(#1375,#761,#762,#763),#8372,.T.);
#8874=ADVANCED_FACE('',(#1376),#8373,.F.);
#8875=ADVANCED_FACE('',(#1377),#8374,.F.);
#8876=ADVANCED_FACE('',(#1378,#764,#765,#766),#8375,.F.);
#8877=ADVANCED_FACE('',(#1379,#767),#946,.F.);
#8878=ADVANCED_FACE('',(#1380,#768),#947,.T.);
#8879=ADVANCED_FACE('',(#1381),#8376,.T.);
#8880=ADVANCED_FACE('',(#1382,#769),#948,.F.);
#8881=ADVANCED_FACE('',(#1383,#770),#949,.F.);
#8882=ADVANCED_FACE('',(#1384),#8377,.T.);
#8883=ADVANCED_FACE('',(#1385,#771),#950,.T.);
#8884=ADVANCED_FACE('',(#1386),#8378,.F.);
#8885=ADVANCED_FACE('',(#1387),#8379,.T.);
#8886=ADVANCED_FACE('',(#1388),#8380,.F.);
#8887=ADVANCED_FACE('',(#1389),#8381,.T.);
#8888=ADVANCED_FACE('',(#1390),#8382,.F.);
#8889=ADVANCED_FACE('',(#1391),#8383,.T.);
#8890=ADVANCED_FACE('',(#1392),#8384,.F.);
#8891=ADVANCED_FACE('',(#1393),#8385,.T.);
#8892=ADVANCED_FACE('',(#1394),#8386,.F.);
#8893=ADVANCED_FACE('',(#1395),#8387,.T.);
#8894=ADVANCED_FACE('',(#1396),#8388,.F.);
#8895=ADVANCED_FACE('',(#1397),#8389,.T.);
#8896=ADVANCED_FACE('',(#1398),#8390,.F.);
#8897=ADVANCED_FACE('',(#1399),#8391,.T.);
#8898=ADVANCED_FACE('',(#1400),#8392,.F.);
#8899=ADVANCED_FACE('',(#1401),#8393,.T.);
#8900=ADVANCED_FACE('',(#1402),#8394,.F.);
#8901=ADVANCED_FACE('',(#1403),#8395,.T.);
#8902=ADVANCED_FACE('',(#1404),#8396,.F.);
#8903=ADVANCED_FACE('',(#1405),#8397,.T.);
#8904=ADVANCED_FACE('',(#1406),#8398,.F.);
#8905=ADVANCED_FACE('',(#1407),#8399,.T.);
#8906=ADVANCED_FACE('',(#1408),#8400,.F.);
#8907=ADVANCED_FACE('',(#1409),#8401,.T.);
#8908=ADVANCED_FACE('',(#1410),#8402,.F.);
#8909=ADVANCED_FACE('',(#1411),#8403,.T.);
#8910=ADVANCED_FACE('',(#1412),#8404,.F.);
#8911=ADVANCED_FACE('',(#1413),#8405,.T.);
#8912=ADVANCED_FACE('',(#1414),#8406,.F.);
#8913=ADVANCED_FACE('',(#1415),#8407,.T.);
#8914=ADVANCED_FACE('',(#1416),#8408,.F.);
#8915=ADVANCED_FACE('',(#1417),#8409,.T.);
#8916=ADVANCED_FACE('',(#1418),#8410,.F.);
#8917=ADVANCED_FACE('',(#1419),#8411,.T.);
#8918=ADVANCED_FACE('',(#1420),#8412,.F.);
#8919=ADVANCED_FACE('',(#1421),#8413,.T.);
#8920=ADVANCED_FACE('',(#1422),#8414,.F.);
#8921=ADVANCED_FACE('',(#1423),#8415,.T.);
#8922=ADVANCED_FACE('',(#1424),#8416,.F.);
#8923=ADVANCED_FACE('',(#1425),#8417,.T.);
#8924=ADVANCED_FACE('',(#1426),#8418,.F.);
#8925=ADVANCED_FACE('',(#1427),#8419,.T.);
#8926=ADVANCED_FACE('',(#1428),#8420,.F.);
#8927=ADVANCED_FACE('',(#1429),#8421,.T.);
#8928=ADVANCED_FACE('',(#1430),#8422,.F.);
#8929=ADVANCED_FACE('',(#1431),#8423,.T.);
#8930=ADVANCED_FACE('',(#1432),#8424,.F.);
#8931=ADVANCED_FACE('',(#1433),#8425,.T.);
#8932=ADVANCED_FACE('',(#1434),#8426,.F.);
#8933=ADVANCED_FACE('',(#1435),#8427,.T.);
#8934=ADVANCED_FACE('',(#1436),#8428,.F.);
#8935=ADVANCED_FACE('',(#1437),#8429,.T.);
#8936=ADVANCED_FACE('',(#1438),#8430,.F.);
#8937=ADVANCED_FACE('',(#1439),#8431,.T.);
#8938=ADVANCED_FACE('',(#1440),#8432,.F.);
#8939=ADVANCED_FACE('',(#1441),#8433,.T.);
#8940=ADVANCED_FACE('',(#1442),#8434,.F.);
#8941=ADVANCED_FACE('',(#1443),#8435,.T.);
#8942=ADVANCED_FACE('',(#1444),#8436,.F.);
#8943=ADVANCED_FACE('',(#1445),#8437,.T.);
#8944=ADVANCED_FACE('',(#1446),#8438,.F.);
#8945=ADVANCED_FACE('',(#1447),#8439,.T.);
#8946=ADVANCED_FACE('',(#1448),#8440,.F.);
#8947=ADVANCED_FACE('',(#1449),#8441,.T.);
#8948=ADVANCED_FACE('',(#1450),#8442,.F.);
#8949=ADVANCED_FACE('',(#1451),#8443,.T.);
#8950=ADVANCED_FACE('',(#1452),#8444,.F.);
#8951=ADVANCED_FACE('',(#1453),#8445,.T.);
#8952=ADVANCED_FACE('',(#1454),#8446,.F.);
#8953=ADVANCED_FACE('',(#1455),#8447,.T.);
#8954=ADVANCED_FACE('',(#1456),#8448,.F.);
#8955=ADVANCED_FACE('',(#1457),#8449,.T.);
#8956=ADVANCED_FACE('',(#1458),#8450,.F.);
#8957=ADVANCED_FACE('',(#1459),#8451,.T.);
#8958=ADVANCED_FACE('',(#1460),#8452,.F.);
#8959=ADVANCED_FACE('',(#1461),#8453,.T.);
#8960=ADVANCED_FACE('',(#1462),#8454,.F.);
#8961=ADVANCED_FACE('',(#1463),#8455,.T.);
#8962=ADVANCED_FACE('',(#1464),#8456,.F.);
#8963=ADVANCED_FACE('',(#1465),#8457,.T.);
#9039=CLOSED_SHELL('',(#8871,#8872,#8873,#8874,#8875,#8876,#8877,#8878,
#8879,#8880,#8881,#8882,#8883,#8884,#8885,#8886,#8887,#8888,#8889,#8890,
#8891,#8892,#8893,#8894,#8895,#8896,#8897,#8898,#8899,#8900,#8901,#8902,
#8903,#8904,#8905,#8906,#8907,#8908,#8909,#8910,#8911,#8912,#8913,#8914,
#8915,#8916,#8917,#8918,#8919,#8920,#8921,#8922,#8923,#8924,#8925,#8926,
#8927,#8928,#8929,#8930,#8931,#8932,#8933,#8934,#8935,#8936,#8937,#8938,
#8939,#8940,#8941,#8942,#8943,#8944,#8945,#8946,#8947,#8948,#8949,#8950,
#8951,#8952,#8953,#8954,#8955,#8956,#8957,#8958,#8959,#8960,#8961,#8962,
#8963));
#10458=AXIS2_PLACEMENT_3D('',#16756,#13057,#13058);
#10459=AXIS2_PLACEMENT_3D('',#16757,#13059,#13060);
#10460=AXIS2_PLACEMENT_3D('',#16844,#13062,#13063);
#10461=AXIS2_PLACEMENT_3D('',#16925,#13065,#13066);
#10462=AXIS2_PLACEMENT_3D('',#16927,#13067,#13068);
#10463=AXIS2_PLACEMENT_3D('',#16931,#13071,#13072);
#10464=AXIS2_PLACEMENT_3D('',#17014,#13073,#13074);
#10465=AXIS2_PLACEMENT_3D('',#17054,#13076,#13077);
#10466=AXIS2_PLACEMENT_3D('',#17094,#13079,#13080);
#10467=AXIS2_PLACEMENT_3D('',#17096,#13081,#13082);
#10468=AXIS2_PLACEMENT_3D('',#17100,#13085,#13086);
#10469=AXIS2_PLACEMENT_3D('',#17101,#13087,#13088);
#10470=AXIS2_PLACEMENT_3D('',#17102,#13089,#13090);
#10471=AXIS2_PLACEMENT_3D('',#17104,#13091,#13092);
#10472=AXIS2_PLACEMENT_3D('',#17107,#13093,#13094);
#10473=AXIS2_PLACEMENT_3D('',#17109,#13095,#13096);
#10474=AXIS2_PLACEMENT_3D('',#17111,#13097,#13098);
#10475=AXIS2_PLACEMENT_3D('',#17113,#13099,#13100);
#10476=AXIS2_PLACEMENT_3D('',#17115,#13101,#13102);
#10477=AXIS2_PLACEMENT_3D('',#17117,#13103,#13104);
#10478=AXIS2_PLACEMENT_3D('',#17119,#13105,#13106);
#10479=AXIS2_PLACEMENT_3D('',#17121,#13107,#13108);
#10480=AXIS2_PLACEMENT_3D('',#17123,#13109,#13110);
#10481=AXIS2_PLACEMENT_3D('',#17125,#13111,#13112);
#10482=AXIS2_PLACEMENT_3D('',#17127,#13113,#13114);
#10483=AXIS2_PLACEMENT_3D('',#17129,#13115,#13116);
#10484=AXIS2_PLACEMENT_3D('',#17131,#13117,#13118);
#10485=AXIS2_PLACEMENT_3D('',#17133,#13119,#13120);
#10486=AXIS2_PLACEMENT_3D('',#17135,#13121,#13122);
#10487=AXIS2_PLACEMENT_3D('',#17137,#13123,#13124);
#10488=AXIS2_PLACEMENT_3D('',#17139,#13125,#13126);
#10489=AXIS2_PLACEMENT_3D('',#17141,#13127,#13128);
#10490=AXIS2_PLACEMENT_3D('',#17143,#13129,#13130);
#10491=AXIS2_PLACEMENT_3D('',#17145,#13131,#13132);
#10492=AXIS2_PLACEMENT_3D('',#17147,#13133,#13134);
#10493=AXIS2_PLACEMENT_3D('',#17149,#13135,#13136);
#10494=AXIS2_PLACEMENT_3D('',#17151,#13137,#13138);
#10495=AXIS2_PLACEMENT_3D('',#17153,#13139,#13140);
#10496=AXIS2_PLACEMENT_3D('',#17155,#13141,#13142);
#10497=AXIS2_PLACEMENT_3D('',#17157,#13143,#13144);
#10498=AXIS2_PLACEMENT_3D('',#17159,#13145,#13146);
#10499=AXIS2_PLACEMENT_3D('',#17161,#13147,#13148);
#10500=AXIS2_PLACEMENT_3D('',#17163,#13149,#13150);
#10501=AXIS2_PLACEMENT_3D('',#17165,#13151,#13152);
#10502=AXIS2_PLACEMENT_3D('',#17167,#13153,#13154);
#10503=AXIS2_PLACEMENT_3D('',#17169,#13155,#13156);
#10504=AXIS2_PLACEMENT_3D('',#17171,#13157,#13158);
#10505=AXIS2_PLACEMENT_3D('',#17173,#13159,#13160);
#10506=AXIS2_PLACEMENT_3D('',#17175,#13161,#13162);
#10507=AXIS2_PLACEMENT_3D('',#17177,#13163,#13164);
#10508=AXIS2_PLACEMENT_3D('',#17179,#13165,#13166);
#10509=AXIS2_PLACEMENT_3D('',#17181,#13167,#13168);
#10510=AXIS2_PLACEMENT_3D('',#17183,#13169,#13170);
#10511=AXIS2_PLACEMENT_3D('',#17185,#13171,#13172);
#10512=AXIS2_PLACEMENT_3D('',#17187,#13173,#13174);
#10513=AXIS2_PLACEMENT_3D('',#17189,#13175,#13176);
#10514=AXIS2_PLACEMENT_3D('',#17191,#13177,#13178);
#10515=AXIS2_PLACEMENT_3D('',#17193,#13179,#13180);
#10516=AXIS2_PLACEMENT_3D('',#17195,#13181,#13182);
#10517=AXIS2_PLACEMENT_3D('',#17197,#13183,#13184);
#10518=AXIS2_PLACEMENT_3D('',#17199,#13185,#13186);
#10519=AXIS2_PLACEMENT_3D('',#17201,#13187,#13188);
#10520=AXIS2_PLACEMENT_3D('',#17203,#13189,#13190);
#10521=AXIS2_PLACEMENT_3D('',#17205,#13191,#13192);
#10522=AXIS2_PLACEMENT_3D('',#17207,#13193,#13194);
#10523=AXIS2_PLACEMENT_3D('',#17209,#13195,#13196);
#10524=AXIS2_PLACEMENT_3D('',#17211,#13197,#13198);
#10525=AXIS2_PLACEMENT_3D('',#17213,#13199,#13200);
#10526=AXIS2_PLACEMENT_3D('',#17215,#13201,#13202);
#10527=AXIS2_PLACEMENT_3D('',#17217,#13203,#13204);
#10528=AXIS2_PLACEMENT_3D('',#17219,#13205,#13206);
#10529=AXIS2_PLACEMENT_3D('',#17221,#13207,#13208);
#10530=AXIS2_PLACEMENT_3D('',#17223,#13209,#13210);
#10531=AXIS2_PLACEMENT_3D('',#17225,#13211,#13212);
#10532=AXIS2_PLACEMENT_3D('',#17227,#13213,#13214);
#10533=AXIS2_PLACEMENT_3D('',#17229,#13215,#13216);
#10534=AXIS2_PLACEMENT_3D('',#17231,#13217,#13218);
#10535=AXIS2_PLACEMENT_3D('',#17233,#13219,#13220);
#10536=AXIS2_PLACEMENT_3D('',#17235,#13221,#13222);
#10537=AXIS2_PLACEMENT_3D('',#17237,#13223,#13224);
#10538=AXIS2_PLACEMENT_3D('',#17239,#13225,#13226);
#10539=AXIS2_PLACEMENT_3D('',#17241,#13227,#13228);
#10540=AXIS2_PLACEMENT_3D('',#17243,#13229,#13230);
#10541=AXIS2_PLACEMENT_3D('',#17245,#13231,#13232);
#10542=AXIS2_PLACEMENT_3D('',#17247,#13233,#13234);
#10543=AXIS2_PLACEMENT_3D('',#17249,#13235,#13236);
#10544=AXIS2_PLACEMENT_3D('',#17251,#13237,#13238);
#10545=AXIS2_PLACEMENT_3D('',#17253,#13239,#13240);
#10546=AXIS2_PLACEMENT_3D('',#17255,#13241,#13242);
#10547=AXIS2_PLACEMENT_3D('',#17257,#13243,#13244);
#10548=AXIS2_PLACEMENT_3D('',#17259,#13245,#13246);
#10549=AXIS2_PLACEMENT_3D('',#17261,#13247,#13248);
#10550=AXIS2_PLACEMENT_3D('',#17263,#13249,#13250);
#10551=AXIS2_PLACEMENT_3D('',#17264,#13251,#13252);
#10552=AXIS2_PLACEMENT_3D('',#17265,#13253,#13254);
#10553=AXIS2_PLACEMENT_3D('',#17267,#13255,#13256);
#10554=AXIS2_PLACEMENT_3D('',#17269,#13258,#13259);
#10555=AXIS2_PLACEMENT_3D('',#17270,#13260,#13261);
#10556=AXIS2_PLACEMENT_3D('',#17272,#13262,#13263);
#10557=AXIS2_PLACEMENT_3D('',#17275,#13264,#13265);
#10558=AXIS2_PLACEMENT_3D('',#17277,#13266,#13267);
#10559=AXIS2_PLACEMENT_3D('',#17279,#13268,#13269);
#10560=AXIS2_PLACEMENT_3D('',#17281,#13270,#13271);
#10561=AXIS2_PLACEMENT_3D('',#17283,#13272,#13273);
#10562=AXIS2_PLACEMENT_3D('',#17285,#13274,#13275);
#10563=AXIS2_PLACEMENT_3D('',#17287,#13276,#13277);
#10564=AXIS2_PLACEMENT_3D('',#17289,#13278,#13279);
#10565=AXIS2_PLACEMENT_3D('',#17291,#13280,#13281);
#10566=AXIS2_PLACEMENT_3D('',#17293,#13282,#13283);
#10567=AXIS2_PLACEMENT_3D('',#17295,#13284,#13285);
#10568=AXIS2_PLACEMENT_3D('',#17297,#13286,#13287);
#10569=AXIS2_PLACEMENT_3D('',#17299,#13288,#13289);
#10570=AXIS2_PLACEMENT_3D('',#17301,#13290,#13291);
#10571=AXIS2_PLACEMENT_3D('',#17303,#13292,#13293);
#10572=AXIS2_PLACEMENT_3D('',#17305,#13294,#13295);
#10573=AXIS2_PLACEMENT_3D('',#17307,#13296,#13297);
#10574=AXIS2_PLACEMENT_3D('',#17309,#13298,#13299);
#10575=AXIS2_PLACEMENT_3D('',#17311,#13300,#13301);
#10576=AXIS2_PLACEMENT_3D('',#17313,#13302,#13303);
#10577=AXIS2_PLACEMENT_3D('',#17315,#13304,#13305);
#10578=AXIS2_PLACEMENT_3D('',#17317,#13306,#13307);
#10579=AXIS2_PLACEMENT_3D('',#17319,#13308,#13309);
#10580=AXIS2_PLACEMENT_3D('',#17321,#13310,#13311);
#10581=AXIS2_PLACEMENT_3D('',#17323,#13312,#13313);
#10582=AXIS2_PLACEMENT_3D('',#17325,#13314,#13315);
#10583=AXIS2_PLACEMENT_3D('',#17327,#13316,#13317);
#10584=AXIS2_PLACEMENT_3D('',#17329,#13318,#13319);
#10585=AXIS2_PLACEMENT_3D('',#17331,#13320,#13321);
#10586=AXIS2_PLACEMENT_3D('',#17333,#13322,#13323);
#10587=AXIS2_PLACEMENT_3D('',#17335,#13324,#13325);
#10588=AXIS2_PLACEMENT_3D('',#17337,#13326,#13327);
#10589=AXIS2_PLACEMENT_3D('',#17339,#13328,#13329);
#10590=AXIS2_PLACEMENT_3D('',#17341,#13330,#13331);
#10591=AXIS2_PLACEMENT_3D('',#17343,#13332,#13333);
#10592=AXIS2_PLACEMENT_3D('',#17345,#13334,#13335);
#10593=AXIS2_PLACEMENT_3D('',#17347,#13336,#13337);
#10594=AXIS2_PLACEMENT_3D('',#17349,#13338,#13339);
#10595=AXIS2_PLACEMENT_3D('',#17351,#13340,#13341);
#10596=AXIS2_PLACEMENT_3D('',#17353,#13342,#13343);
#10597=AXIS2_PLACEMENT_3D('',#17355,#13344,#13345);
#10598=AXIS2_PLACEMENT_3D('',#17357,#13346,#13347);
#10599=AXIS2_PLACEMENT_3D('',#17359,#13348,#13349);
#10600=AXIS2_PLACEMENT_3D('',#17361,#13350,#13351);
#10601=AXIS2_PLACEMENT_3D('',#17363,#13352,#13353);
#10602=AXIS2_PLACEMENT_3D('',#17365,#13354,#13355);
#10603=AXIS2_PLACEMENT_3D('',#17367,#13356,#13357);
#10604=AXIS2_PLACEMENT_3D('',#17369,#13358,#13359);
#10605=AXIS2_PLACEMENT_3D('',#17371,#13360,#13361);
#10606=AXIS2_PLACEMENT_3D('',#17373,#13362,#13363);
#10607=AXIS2_PLACEMENT_3D('',#17375,#13364,#13365);
#10608=AXIS2_PLACEMENT_3D('',#17377,#13366,#13367);
#10609=AXIS2_PLACEMENT_3D('',#17379,#13368,#13369);
#10610=AXIS2_PLACEMENT_3D('',#17381,#13370,#13371);
#10611=AXIS2_PLACEMENT_3D('',#17383,#13372,#13373);
#10612=AXIS2_PLACEMENT_3D('',#17385,#13374,#13375);
#10613=AXIS2_PLACEMENT_3D('',#17387,#13376,#13377);
#10614=AXIS2_PLACEMENT_3D('',#17389,#13378,#13379);
#10615=AXIS2_PLACEMENT_3D('',#17391,#13380,#13381);
#10616=AXIS2_PLACEMENT_3D('',#17393,#13382,#13383);
#10617=AXIS2_PLACEMENT_3D('',#17395,#13384,#13385);
#10618=AXIS2_PLACEMENT_3D('',#17397,#13386,#13387);
#10619=AXIS2_PLACEMENT_3D('',#17399,#13388,#13389);
#10620=AXIS2_PLACEMENT_3D('',#17401,#13390,#13391);
#10621=AXIS2_PLACEMENT_3D('',#17403,#13392,#13393);
#10622=AXIS2_PLACEMENT_3D('',#17405,#13394,#13395);
#10623=AXIS2_PLACEMENT_3D('',#17407,#13396,#13397);
#10624=AXIS2_PLACEMENT_3D('',#17409,#13398,#13399);
#10625=AXIS2_PLACEMENT_3D('',#17411,#13400,#13401);
#10626=AXIS2_PLACEMENT_3D('',#17413,#13402,#13403);
#10627=AXIS2_PLACEMENT_3D('',#17415,#13404,#13405);
#10628=AXIS2_PLACEMENT_3D('',#17417,#13406,#13407);
#10629=AXIS2_PLACEMENT_3D('',#17419,#13408,#13409);
#10630=AXIS2_PLACEMENT_3D('',#17421,#13410,#13411);
#10631=AXIS2_PLACEMENT_3D('',#17423,#13412,#13413);
#10632=AXIS2_PLACEMENT_3D('',#17425,#13414,#13415);
#10633=AXIS2_PLACEMENT_3D('',#17427,#13416,#13417);
#10634=AXIS2_PLACEMENT_3D('',#17429,#13418,#13419);
#10635=AXIS2_PLACEMENT_3D('',#17431,#13420,#13421);
#10636=AXIS2_PLACEMENT_3D('',#17432,#13422,#13423);
#10637=AXIS2_PLACEMENT_3D('',#17433,#13424,#13425);
#10638=AXIS2_PLACEMENT_3D('',#17435,#13426,#13427);
#10639=AXIS2_PLACEMENT_3D('',#17437,#13429,#13430);
#10640=AXIS2_PLACEMENT_3D('',#17438,#13431,#13432);
#10641=AXIS2_PLACEMENT_3D('',#17441,#13435,#13436);
#10642=AXIS2_PLACEMENT_3D('',#17443,#13438,#13439);
#10643=AXIS2_PLACEMENT_3D('',#17445,#13441,#13442);
#10644=AXIS2_PLACEMENT_3D('',#17447,#13444,#13445);
#10645=AXIS2_PLACEMENT_3D('',#17449,#13447,#13448);
#10646=AXIS2_PLACEMENT_3D('',#17451,#13450,#13451);
#10647=AXIS2_PLACEMENT_3D('',#17453,#13453,#13454);
#10648=AXIS2_PLACEMENT_3D('',#17455,#13456,#13457);
#10649=AXIS2_PLACEMENT_3D('',#17457,#13459,#13460);
#10650=AXIS2_PLACEMENT_3D('',#17459,#13462,#13463);
#10651=AXIS2_PLACEMENT_3D('',#17461,#13465,#13466);
#10652=AXIS2_PLACEMENT_3D('',#17463,#13468,#13469);
#10653=AXIS2_PLACEMENT_3D('',#17465,#13471,#13472);
#10654=AXIS2_PLACEMENT_3D('',#17467,#13474,#13475);
#10655=AXIS2_PLACEMENT_3D('',#17469,#13477,#13478);
#10656=AXIS2_PLACEMENT_3D('',#17471,#13480,#13481);
#10657=AXIS2_PLACEMENT_3D('',#17473,#13483,#13484);
#10658=AXIS2_PLACEMENT_3D('',#17475,#13486,#13487);
#10659=AXIS2_PLACEMENT_3D('',#17477,#13489,#13490);
#10660=AXIS2_PLACEMENT_3D('',#17479,#13492,#13493);
#10661=AXIS2_PLACEMENT_3D('',#17481,#13495,#13496);
#10662=AXIS2_PLACEMENT_3D('',#17483,#13498,#13499);
#10663=AXIS2_PLACEMENT_3D('',#17485,#13501,#13502);
#10664=AXIS2_PLACEMENT_3D('',#17487,#13504,#13505);
#10665=AXIS2_PLACEMENT_3D('',#17489,#13507,#13508);
#10666=AXIS2_PLACEMENT_3D('',#17491,#13510,#13511);
#10667=AXIS2_PLACEMENT_3D('',#17493,#13513,#13514);
#10668=AXIS2_PLACEMENT_3D('',#17495,#13516,#13517);
#10669=AXIS2_PLACEMENT_3D('',#17497,#13519,#13520);
#10670=AXIS2_PLACEMENT_3D('',#17499,#13522,#13523);
#10671=AXIS2_PLACEMENT_3D('',#17501,#13525,#13526);
#10672=AXIS2_PLACEMENT_3D('',#17503,#13528,#13529);
#10673=AXIS2_PLACEMENT_3D('',#17505,#13531,#13532);
#10674=AXIS2_PLACEMENT_3D('',#17507,#13534,#13535);
#10675=AXIS2_PLACEMENT_3D('',#17509,#13537,#13538);
#10676=AXIS2_PLACEMENT_3D('',#17511,#13540,#13541);
#10677=AXIS2_PLACEMENT_3D('',#17513,#13543,#13544);
#10678=AXIS2_PLACEMENT_3D('',#17515,#13546,#13547);
#10679=AXIS2_PLACEMENT_3D('',#17517,#13549,#13550);
#10680=AXIS2_PLACEMENT_3D('',#17519,#13552,#13553);
#10681=AXIS2_PLACEMENT_3D('',#17521,#13555,#13556);
#10682=AXIS2_PLACEMENT_3D('',#17523,#13558,#13559);
#10683=AXIS2_PLACEMENT_3D('',#17525,#13561,#13562);
#10684=AXIS2_PLACEMENT_3D('',#17527,#13564,#13565);
#10685=AXIS2_PLACEMENT_3D('',#17529,#13567,#13568);
#10686=AXIS2_PLACEMENT_3D('',#17531,#13570,#13571);
#10687=AXIS2_PLACEMENT_3D('',#17533,#13573,#13574);
#10688=AXIS2_PLACEMENT_3D('',#17535,#13576,#13577);
#10689=AXIS2_PLACEMENT_3D('',#17537,#13579,#13580);
#10690=AXIS2_PLACEMENT_3D('',#17539,#13582,#13583);
#10691=AXIS2_PLACEMENT_3D('',#17541,#13585,#13586);
#10692=AXIS2_PLACEMENT_3D('',#17543,#13588,#13589);
#10693=AXIS2_PLACEMENT_3D('',#17545,#13591,#13592);
#10694=AXIS2_PLACEMENT_3D('',#17547,#13594,#13595);
#10695=AXIS2_PLACEMENT_3D('',#17549,#13597,#13598);
#10696=AXIS2_PLACEMENT_3D('',#17551,#13600,#13601);
#10697=AXIS2_PLACEMENT_3D('',#17553,#13603,#13604);
#10698=AXIS2_PLACEMENT_3D('',#17555,#13606,#13607);
#10699=AXIS2_PLACEMENT_3D('',#17557,#13609,#13610);
#10700=AXIS2_PLACEMENT_3D('',#17559,#13612,#13613);
#10701=AXIS2_PLACEMENT_3D('',#17561,#13615,#13616);
#10702=AXIS2_PLACEMENT_3D('',#17563,#13618,#13619);
#10703=AXIS2_PLACEMENT_3D('',#17565,#13621,#13622);
#10704=AXIS2_PLACEMENT_3D('',#17567,#13624,#13625);
#10705=AXIS2_PLACEMENT_3D('',#17569,#13627,#13628);
#10706=AXIS2_PLACEMENT_3D('',#17571,#13630,#13631);
#10707=AXIS2_PLACEMENT_3D('',#17573,#13633,#13634);
#10708=AXIS2_PLACEMENT_3D('',#17575,#13636,#13637);
#10709=AXIS2_PLACEMENT_3D('',#17577,#13639,#13640);
#10710=AXIS2_PLACEMENT_3D('',#17579,#13642,#13643);
#10711=AXIS2_PLACEMENT_3D('',#17581,#13645,#13646);
#10712=AXIS2_PLACEMENT_3D('',#17583,#13648,#13649);
#10713=AXIS2_PLACEMENT_3D('',#17585,#13651,#13652);
#10714=AXIS2_PLACEMENT_3D('',#17587,#13654,#13655);
#10715=AXIS2_PLACEMENT_3D('',#17589,#13657,#13658);
#10716=AXIS2_PLACEMENT_3D('',#17591,#13660,#13661);
#10717=AXIS2_PLACEMENT_3D('',#17593,#13663,#13664);
#10718=AXIS2_PLACEMENT_3D('',#17595,#13666,#13667);
#10719=AXIS2_PLACEMENT_3D('',#17597,#13669,#13670);
#13057=DIRECTION('axis',(0.,0.,1.));
#13058=DIRECTION('refdir',(1.,0.,0.));
#13059=DIRECTION('center_axis',(1.,0.,6.12323399573677E-17));
#13060=DIRECTION('ref_axis',(6.12323399573677E-17,0.,-1.));
#13061=DIRECTION('',(1.,0.,6.12323399573677E-17));
#13062=DIRECTION('center_axis',(1.,0.,6.12323399573677E-17));
#13063=DIRECTION('ref_axis',(6.12323399573677E-17,0.,-1.));
#13064=DIRECTION('',(1.,0.,6.12323399573677E-17));
#13065=DIRECTION('center_axis',(0.,-1.,0.));
#13066=DIRECTION('ref_axis',(1.,0.,0.));
#13067=DIRECTION('center_axis',(0.,-1.,0.));
#13068=DIRECTION('ref_axis',(1.,0.,0.));
#13069=DIRECTION('',(0.,1.,0.));
#13070=DIRECTION('',(0.,1.,0.));
#13071=DIRECTION('center_axis',(0.,1.,0.));
#13072=DIRECTION('ref_axis',(1.,0.,0.));
#13073=DIRECTION('center_axis',(0.,0.,1.));
#13074=DIRECTION('ref_axis',(1.,0.,0.));
#13075=DIRECTION('',(0.,0.,1.));
#13076=DIRECTION('center_axis',(0.,0.,1.));
#13077=DIRECTION('ref_axis',(1.,0.,0.));
#13078=DIRECTION('',(0.,0.,1.));
#13079=DIRECTION('center_axis',(0.,1.,0.));
#13080=DIRECTION('ref_axis',(1.,0.,0.));
#13081=DIRECTION('center_axis',(0.,1.,0.));
#13082=DIRECTION('ref_axis',(1.,0.,0.));
#13083=DIRECTION('',(0.,1.,0.));
#13084=DIRECTION('',(0.,1.,0.));
#13085=DIRECTION('center_axis',(0.,-1.,0.));
#13086=DIRECTION('ref_axis',(1.,0.,0.));
#13087=DIRECTION('center_axis',(0.,1.,0.));
#13088=DIRECTION('ref_axis',(1.,0.,0.));
#13089=DIRECTION('center_axis',(0.,1.,0.));
#13090=DIRECTION('ref_axis',(1.,0.,0.));
#13091=DIRECTION('center_axis',(0.,1.,0.));
#13092=DIRECTION('ref_axis',(1.,0.,0.));
#13093=DIRECTION('center_axis',(0.,1.,0.));
#13094=DIRECTION('ref_axis',(0.987688340595138,0.,0.156434465040231));
#13095=DIRECTION('center_axis',(0.,1.,0.));
#13096=DIRECTION('ref_axis',(1.,0.,0.));
#13097=DIRECTION('center_axis',(0.,1.,0.));
#13098=DIRECTION('ref_axis',(0.951056516295154,0.,0.309016994374948));
#13099=DIRECTION('center_axis',(0.,1.,0.));
#13100=DIRECTION('ref_axis',(1.,0.,0.));
#13101=DIRECTION('center_axis',(0.,1.,0.));
#13102=DIRECTION('ref_axis',(0.891006524188368,0.,0.453990499739547));
#13103=DIRECTION('center_axis',(0.,1.,0.));
#13104=DIRECTION('ref_axis',(1.,0.,0.));
#13105=DIRECTION('center_axis',(0.,1.,0.));
#13106=DIRECTION('ref_axis',(0.809016994374947,0.,0.587785252292473));
#13107=DIRECTION('center_axis',(0.,1.,0.));
#13108=DIRECTION('ref_axis',(1.,0.,0.));
#13109=DIRECTION('center_axis',(0.,1.,0.));
#13110=DIRECTION('ref_axis',(0.707106781186547,0.,0.707106781186548));
#13111=DIRECTION('center_axis',(0.,1.,0.));
#13112=DIRECTION('ref_axis',(1.,0.,0.));
#13113=DIRECTION('center_axis',(0.,1.,0.));
#13114=DIRECTION('ref_axis',(0.587785252292473,0.,0.809016994374948));
#13115=DIRECTION('center_axis',(0.,1.,0.));
#13116=DIRECTION('ref_axis',(1.,0.,0.));
#13117=DIRECTION('center_axis',(0.,1.,0.));
#13118=DIRECTION('ref_axis',(0.453990499739547,0.,0.891006524188368));
#13119=DIRECTION('center_axis',(0.,1.,0.));
#13120=DIRECTION('ref_axis',(1.,0.,0.));
#13121=DIRECTION('center_axis',(0.,1.,0.));
#13122=DIRECTION('ref_axis',(0.309016994374947,0.,0.951056516295154));
#13123=DIRECTION('center_axis',(0.,1.,0.));
#13124=DIRECTION('ref_axis',(1.,0.,0.));
#13125=DIRECTION('center_axis',(0.,1.,0.));
#13126=DIRECTION('ref_axis',(0.156434465040231,0.,0.987688340595138));
#13127=DIRECTION('center_axis',(0.,1.,0.));
#13128=DIRECTION('ref_axis',(1.,0.,0.));
#13129=DIRECTION('center_axis',(0.,1.,0.));
#13130=DIRECTION('ref_axis',(-1.83697019872103E-16,0.,1.));
#13131=DIRECTION('center_axis',(0.,1.,0.));
#13132=DIRECTION('ref_axis',(1.,0.,0.));
#13133=DIRECTION('center_axis',(0.,1.,0.));
#13134=DIRECTION('ref_axis',(-0.156434465040231,0.,0.987688340595138));
#13135=DIRECTION('center_axis',(0.,1.,0.));
#13136=DIRECTION('ref_axis',(1.,0.,0.));
#13137=DIRECTION('center_axis',(0.,1.,0.));
#13138=DIRECTION('ref_axis',(-0.309016994374948,0.,0.951056516295154));
#13139=DIRECTION('center_axis',(0.,1.,0.));
#13140=DIRECTION('ref_axis',(1.,0.,0.));
#13141=DIRECTION('center_axis',(0.,1.,0.));
#13142=DIRECTION('ref_axis',(-0.453990499739547,0.,0.891006524188368));
#13143=DIRECTION('center_axis',(0.,1.,0.));
#13144=DIRECTION('ref_axis',(1.,0.,0.));
#13145=DIRECTION('center_axis',(0.,1.,0.));
#13146=DIRECTION('ref_axis',(-0.587785252292473,0.,0.809016994374947));
#13147=DIRECTION('center_axis',(0.,1.,0.));
#13148=DIRECTION('ref_axis',(1.,0.,0.));
#13149=DIRECTION('center_axis',(0.,1.,0.));
#13150=DIRECTION('ref_axis',(-0.707106781186548,0.,0.707106781186547));
#13151=DIRECTION('center_axis',(0.,1.,0.));
#13152=DIRECTION('ref_axis',(1.,0.,0.));
#13153=DIRECTION('center_axis',(0.,1.,0.));
#13154=DIRECTION('ref_axis',(-0.809016994374947,0.,0.587785252292473));
#13155=DIRECTION('center_axis',(0.,1.,0.));
#13156=DIRECTION('ref_axis',(1.,0.,0.));
#13157=DIRECTION('center_axis',(0.,1.,0.));
#13158=DIRECTION('ref_axis',(-0.891006524188368,0.,0.453990499739547));
#13159=DIRECTION('center_axis',(0.,1.,0.));
#13160=DIRECTION('ref_axis',(1.,0.,0.));
#13161=DIRECTION('center_axis',(0.,1.,0.));
#13162=DIRECTION('ref_axis',(-0.951056516295154,0.,0.309016994374947));
#13163=DIRECTION('center_axis',(0.,1.,0.));
#13164=DIRECTION('ref_axis',(1.,0.,0.));
#13165=DIRECTION('center_axis',(0.,1.,0.));
#13166=DIRECTION('ref_axis',(-0.987688340595138,0.,0.156434465040231));
#13167=DIRECTION('center_axis',(0.,1.,0.));
#13168=DIRECTION('ref_axis',(1.,0.,0.));
#13169=DIRECTION('center_axis',(0.,1.,0.));
#13170=DIRECTION('ref_axis',(-1.,0.,-1.22464679914735E-16));
#13171=DIRECTION('center_axis',(0.,1.,0.));
#13172=DIRECTION('ref_axis',(1.,0.,0.));
#13173=DIRECTION('center_axis',(0.,1.,0.));
#13174=DIRECTION('ref_axis',(-0.987688340595138,0.,-0.156434465040231));
#13175=DIRECTION('center_axis',(0.,1.,0.));
#13176=DIRECTION('ref_axis',(1.,0.,0.));
#13177=DIRECTION('center_axis',(0.,1.,0.));
#13178=DIRECTION('ref_axis',(-0.951056516295154,0.,-0.309016994374948));
#13179=DIRECTION('center_axis',(0.,1.,0.));
#13180=DIRECTION('ref_axis',(1.,0.,0.));
#13181=DIRECTION('center_axis',(0.,1.,0.));
#13182=DIRECTION('ref_axis',(-0.891006524188368,0.,-0.453990499739547));
#13183=DIRECTION('center_axis',(0.,1.,0.));
#13184=DIRECTION('ref_axis',(1.,0.,0.));
#13185=DIRECTION('center_axis',(0.,1.,0.));
#13186=DIRECTION('ref_axis',(-0.809016994374947,0.,-0.587785252292473));
#13187=DIRECTION('center_axis',(0.,1.,0.));
#13188=DIRECTION('ref_axis',(1.,0.,0.));
#13189=DIRECTION('center_axis',(0.,1.,0.));
#13190=DIRECTION('ref_axis',(-0.707106781186547,0.,-0.707106781186548));
#13191=DIRECTION('center_axis',(0.,1.,0.));
#13192=DIRECTION('ref_axis',(1.,0.,0.));
#13193=DIRECTION('center_axis',(0.,1.,0.));
#13194=DIRECTION('ref_axis',(-0.587785252292473,0.,-0.809016994374947));
#13195=DIRECTION('center_axis',(0.,1.,0.));
#13196=DIRECTION('ref_axis',(1.,0.,0.));
#13197=DIRECTION('center_axis',(0.,1.,0.));
#13198=DIRECTION('ref_axis',(-0.453990499739547,0.,-0.891006524188368));
#13199=DIRECTION('center_axis',(0.,1.,0.));
#13200=DIRECTION('ref_axis',(1.,0.,0.));
#13201=DIRECTION('center_axis',(0.,1.,0.));
#13202=DIRECTION('ref_axis',(-0.309016994374947,0.,-0.951056516295154));
#13203=DIRECTION('center_axis',(0.,1.,0.));
#13204=DIRECTION('ref_axis',(1.,0.,0.));
#13205=DIRECTION('center_axis',(0.,1.,0.));
#13206=DIRECTION('ref_axis',(-0.156434465040231,0.,-0.987688340595138));
#13207=DIRECTION('center_axis',(0.,1.,0.));
#13208=DIRECTION('ref_axis',(1.,0.,0.));
#13209=DIRECTION('center_axis',(0.,1.,0.));
#13210=DIRECTION('ref_axis',(6.12323399573677E-17,0.,-1.));
#13211=DIRECTION('center_axis',(0.,1.,0.));
#13212=DIRECTION('ref_axis',(1.,0.,0.));
#13213=DIRECTION('center_axis',(0.,1.,0.));
#13214=DIRECTION('ref_axis',(0.156434465040231,0.,-0.987688340595138));
#13215=DIRECTION('center_axis',(0.,1.,0.));
#13216=DIRECTION('ref_axis',(1.,0.,0.));
#13217=DIRECTION('center_axis',(0.,1.,0.));
#13218=DIRECTION('ref_axis',(0.309016994374948,0.,-0.951056516295154));
#13219=DIRECTION('center_axis',(0.,1.,0.));
#13220=DIRECTION('ref_axis',(1.,0.,0.));
#13221=DIRECTION('center_axis',(0.,1.,0.));
#13222=DIRECTION('ref_axis',(0.453990499739547,0.,-0.891006524188368));
#13223=DIRECTION('center_axis',(0.,1.,0.));
#13224=DIRECTION('ref_axis',(1.,0.,0.));
#13225=DIRECTION('center_axis',(0.,1.,0.));
#13226=DIRECTION('ref_axis',(0.587785252292473,0.,-0.809016994374947));
#13227=DIRECTION('center_axis',(0.,1.,0.));
#13228=DIRECTION('ref_axis',(1.,0.,0.));
#13229=DIRECTION('center_axis',(0.,1.,0.));
#13230=DIRECTION('ref_axis',(0.707106781186548,0.,-0.707106781186547));
#13231=DIRECTION('center_axis',(0.,1.,0.));
#13232=DIRECTION('ref_axis',(1.,0.,0.));
#13233=DIRECTION('center_axis',(0.,1.,0.));
#13234=DIRECTION('ref_axis',(0.809016994374947,0.,-0.587785252292473));
#13235=DIRECTION('center_axis',(0.,1.,0.));
#13236=DIRECTION('ref_axis',(1.,0.,0.));
#13237=DIRECTION('center_axis',(0.,1.,0.));
#13238=DIRECTION('ref_axis',(0.891006524188368,0.,-0.453990499739547));
#13239=DIRECTION('center_axis',(0.,1.,0.));
#13240=DIRECTION('ref_axis',(1.,0.,0.));
#13241=DIRECTION('center_axis',(0.,1.,0.));
#13242=DIRECTION('ref_axis',(0.951056516295154,0.,-0.309016994374947));
#13243=DIRECTION('center_axis',(0.,1.,0.));
#13244=DIRECTION('ref_axis',(1.,0.,0.));
#13245=DIRECTION('center_axis',(0.,1.,0.));
#13246=DIRECTION('ref_axis',(0.987688340595138,0.,-0.156434465040231));
#13247=DIRECTION('center_axis',(0.,1.,0.));
#13248=DIRECTION('ref_axis',(1.,0.,0.));
#13249=DIRECTION('center_axis',(0.,1.,0.));
#13250=DIRECTION('ref_axis',(1.,0.,0.));
#13251=DIRECTION('center_axis',(0.,1.,0.));
#13252=DIRECTION('ref_axis',(1.,0.,0.));
#13253=DIRECTION('center_axis',(0.,-1.,0.));
#13254=DIRECTION('ref_axis',(1.,0.,0.));
#13255=DIRECTION('center_axis',(0.,-1.,0.));
#13256=DIRECTION('ref_axis',(1.,0.,0.));
#13257=DIRECTION('',(0.,1.,0.));
#13258=DIRECTION('center_axis',(0.,1.,0.));
#13259=DIRECTION('ref_axis',(1.,0.,0.));
#13260=DIRECTION('center_axis',(0.,1.,0.));
#13261=DIRECTION('ref_axis',(1.,0.,0.));
#13262=DIRECTION('center_axis',(0.,1.,0.));
#13263=DIRECTION('ref_axis',(1.,0.,0.));
#13264=DIRECTION('center_axis',(0.,-1.,0.));
#13265=DIRECTION('ref_axis',(0.987688340595138,0.,0.156434465040231));
#13266=DIRECTION('center_axis',(0.,1.,0.));
#13267=DIRECTION('ref_axis',(1.,0.,0.));
#13268=DIRECTION('center_axis',(0.,-1.,0.));
#13269=DIRECTION('ref_axis',(1.,0.,0.));
#13270=DIRECTION('center_axis',(0.,1.,0.));
#13271=DIRECTION('ref_axis',(1.,0.,0.));
#13272=DIRECTION('center_axis',(0.,-1.,0.));
#13273=DIRECTION('ref_axis',(0.987688340595138,0.,-0.156434465040231));
#13274=DIRECTION('center_axis',(0.,1.,0.));
#13275=DIRECTION('ref_axis',(1.,0.,0.));
#13276=DIRECTION('center_axis',(0.,-1.,0.));
#13277=DIRECTION('ref_axis',(0.951056516295154,0.,-0.309016994374947));
#13278=DIRECTION('center_axis',(0.,1.,0.));
#13279=DIRECTION('ref_axis',(1.,0.,0.));
#13280=DIRECTION('center_axis',(0.,-1.,0.));
#13281=DIRECTION('ref_axis',(0.891006524188368,0.,-0.453990499739547));
#13282=DIRECTION('center_axis',(0.,1.,0.));
#13283=DIRECTION('ref_axis',(1.,0.,0.));
#13284=DIRECTION('center_axis',(0.,-1.,0.));
#13285=DIRECTION('ref_axis',(0.809016994374947,0.,-0.587785252292473));
#13286=DIRECTION('center_axis',(0.,1.,0.));
#13287=DIRECTION('ref_axis',(1.,0.,0.));
#13288=DIRECTION('center_axis',(0.,-1.,0.));
#13289=DIRECTION('ref_axis',(0.707106781186548,0.,-0.707106781186547));
#13290=DIRECTION('center_axis',(0.,1.,0.));
#13291=DIRECTION('ref_axis',(1.,0.,0.));
#13292=DIRECTION('center_axis',(0.,-1.,0.));
#13293=DIRECTION('ref_axis',(0.587785252292473,0.,-0.809016994374947));
#13294=DIRECTION('center_axis',(0.,1.,0.));
#13295=DIRECTION('ref_axis',(1.,0.,0.));
#13296=DIRECTION('center_axis',(0.,-1.,0.));
#13297=DIRECTION('ref_axis',(0.453990499739547,0.,-0.891006524188368));
#13298=DIRECTION('center_axis',(0.,1.,0.));
#13299=DIRECTION('ref_axis',(1.,0.,0.));
#13300=DIRECTION('center_axis',(0.,-1.,0.));
#13301=DIRECTION('ref_axis',(0.309016994374948,0.,-0.951056516295154));
#13302=DIRECTION('center_axis',(0.,1.,0.));
#13303=DIRECTION('ref_axis',(1.,0.,0.));
#13304=DIRECTION('center_axis',(0.,-1.,0.));
#13305=DIRECTION('ref_axis',(0.156434465040231,0.,-0.987688340595138));
#13306=DIRECTION('center_axis',(0.,1.,0.));
#13307=DIRECTION('ref_axis',(1.,0.,0.));
#13308=DIRECTION('center_axis',(0.,-1.,0.));
#13309=DIRECTION('ref_axis',(6.12323399573677E-17,0.,-1.));
#13310=DIRECTION('center_axis',(0.,1.,0.));
#13311=DIRECTION('ref_axis',(1.,0.,0.));
#13312=DIRECTION('center_axis',(0.,-1.,0.));
#13313=DIRECTION('ref_axis',(-0.156434465040231,0.,-0.987688340595138));
#13314=DIRECTION('center_axis',(0.,1.,0.));
#13315=DIRECTION('ref_axis',(1.,0.,0.));
#13316=DIRECTION('center_axis',(0.,-1.,0.));
#13317=DIRECTION('ref_axis',(-0.309016994374947,0.,-0.951056516295154));
#13318=DIRECTION('center_axis',(0.,1.,0.));
#13319=DIRECTION('ref_axis',(1.,0.,0.));
#13320=DIRECTION('center_axis',(0.,-1.,0.));
#13321=DIRECTION('ref_axis',(-0.453990499739547,0.,-0.891006524188368));
#13322=DIRECTION('center_axis',(0.,1.,0.));
#13323=DIRECTION('ref_axis',(1.,0.,0.));
#13324=DIRECTION('center_axis',(0.,-1.,0.));
#13325=DIRECTION('ref_axis',(-0.587785252292473,0.,-0.809016994374947));
#13326=DIRECTION('center_axis',(0.,1.,0.));
#13327=DIRECTION('ref_axis',(1.,0.,0.));
#13328=DIRECTION('center_axis',(0.,-1.,0.));
#13329=DIRECTION('ref_axis',(-0.707106781186547,0.,-0.707106781186548));
#13330=DIRECTION('center_axis',(0.,1.,0.));
#13331=DIRECTION('ref_axis',(1.,0.,0.));
#13332=DIRECTION('center_axis',(0.,-1.,0.));
#13333=DIRECTION('ref_axis',(-0.809016994374947,0.,-0.587785252292473));
#13334=DIRECTION('center_axis',(0.,1.,0.));
#13335=DIRECTION('ref_axis',(1.,0.,0.));
#13336=DIRECTION('center_axis',(0.,-1.,0.));
#13337=DIRECTION('ref_axis',(-0.891006524188368,0.,-0.453990499739547));
#13338=DIRECTION('center_axis',(0.,1.,0.));
#13339=DIRECTION('ref_axis',(1.,0.,0.));
#13340=DIRECTION('center_axis',(0.,-1.,0.));
#13341=DIRECTION('ref_axis',(-0.951056516295154,0.,-0.309016994374948));
#13342=DIRECTION('center_axis',(0.,1.,0.));
#13343=DIRECTION('ref_axis',(1.,0.,0.));
#13344=DIRECTION('center_axis',(0.,-1.,0.));
#13345=DIRECTION('ref_axis',(-0.987688340595138,0.,-0.156434465040231));
#13346=DIRECTION('center_axis',(0.,1.,0.));
#13347=DIRECTION('ref_axis',(1.,0.,0.));
#13348=DIRECTION('center_axis',(0.,-1.,0.));
#13349=DIRECTION('ref_axis',(-1.,0.,-1.22464679914735E-16));
#13350=DIRECTION('center_axis',(0.,1.,0.));
#13351=DIRECTION('ref_axis',(1.,0.,0.));
#13352=DIRECTION('center_axis',(0.,-1.,0.));
#13353=DIRECTION('ref_axis',(-0.987688340595138,0.,0.156434465040231));
#13354=DIRECTION('center_axis',(0.,1.,0.));
#13355=DIRECTION('ref_axis',(1.,0.,0.));
#13356=DIRECTION('center_axis',(0.,-1.,0.));
#13357=DIRECTION('ref_axis',(-0.951056516295154,0.,0.309016994374947));
#13358=DIRECTION('center_axis',(0.,1.,0.));
#13359=DIRECTION('ref_axis',(1.,0.,0.));
#13360=DIRECTION('center_axis',(0.,-1.,0.));
#13361=DIRECTION('ref_axis',(-0.891006524188368,0.,0.453990499739547));
#13362=DIRECTION('center_axis',(0.,1.,0.));
#13363=DIRECTION('ref_axis',(1.,0.,0.));
#13364=DIRECTION('center_axis',(0.,-1.,0.));
#13365=DIRECTION('ref_axis',(-0.809016994374947,0.,0.587785252292473));
#13366=DIRECTION('center_axis',(0.,1.,0.));
#13367=DIRECTION('ref_axis',(1.,0.,0.));
#13368=DIRECTION('center_axis',(0.,-1.,0.));
#13369=DIRECTION('ref_axis',(-0.707106781186548,0.,0.707106781186547));
#13370=DIRECTION('center_axis',(0.,1.,0.));
#13371=DIRECTION('ref_axis',(1.,0.,0.));
#13372=DIRECTION('center_axis',(0.,-1.,0.));
#13373=DIRECTION('ref_axis',(-0.587785252292473,0.,0.809016994374947));
#13374=DIRECTION('center_axis',(0.,1.,0.));
#13375=DIRECTION('ref_axis',(1.,0.,0.));
#13376=DIRECTION('center_axis',(0.,-1.,0.));
#13377=DIRECTION('ref_axis',(-0.453990499739547,0.,0.891006524188368));
#13378=DIRECTION('center_axis',(0.,1.,0.));
#13379=DIRECTION('ref_axis',(1.,0.,0.));
#13380=DIRECTION('center_axis',(0.,-1.,0.));
#13381=DIRECTION('ref_axis',(-0.309016994374948,0.,0.951056516295154));
#13382=DIRECTION('center_axis',(0.,1.,0.));
#13383=DIRECTION('ref_axis',(1.,0.,0.));
#13384=DIRECTION('center_axis',(0.,-1.,0.));
#13385=DIRECTION('ref_axis',(-0.156434465040231,0.,0.987688340595138));
#13386=DIRECTION('center_axis',(0.,1.,0.));
#13387=DIRECTION('ref_axis',(1.,0.,0.));
#13388=DIRECTION('center_axis',(0.,-1.,0.));
#13389=DIRECTION('ref_axis',(-1.83697019872103E-16,0.,1.));
#13390=DIRECTION('center_axis',(0.,1.,0.));
#13391=DIRECTION('ref_axis',(1.,0.,0.));
#13392=DIRECTION('center_axis',(0.,-1.,0.));
#13393=DIRECTION('ref_axis',(0.156434465040231,0.,0.987688340595138));
#13394=DIRECTION('center_axis',(0.,1.,0.));
#13395=DIRECTION('ref_axis',(1.,0.,0.));
#13396=DIRECTION('center_axis',(0.,-1.,0.));
#13397=DIRECTION('ref_axis',(0.309016994374947,0.,0.951056516295154));
#13398=DIRECTION('center_axis',(0.,1.,0.));
#13399=DIRECTION('ref_axis',(1.,0.,0.));
#13400=DIRECTION('center_axis',(0.,-1.,0.));
#13401=DIRECTION('ref_axis',(0.453990499739547,0.,0.891006524188368));
#13402=DIRECTION('center_axis',(0.,1.,0.));
#13403=DIRECTION('ref_axis',(1.,0.,0.));
#13404=DIRECTION('center_axis',(0.,-1.,0.));
#13405=DIRECTION('ref_axis',(0.587785252292473,0.,0.809016994374948));
#13406=DIRECTION('center_axis',(0.,1.,0.));
#13407=DIRECTION('ref_axis',(1.,0.,0.));
#13408=DIRECTION('center_axis',(0.,-1.,0.));
#13409=DIRECTION('ref_axis',(0.707106781186547,0.,0.707106781186548));
#13410=DIRECTION('center_axis',(0.,1.,0.));
#13411=DIRECTION('ref_axis',(1.,0.,0.));
#13412=DIRECTION('center_axis',(0.,-1.,0.));
#13413=DIRECTION('ref_axis',(0.809016994374947,0.,0.587785252292473));
#13414=DIRECTION('center_axis',(0.,1.,0.));
#13415=DIRECTION('ref_axis',(1.,0.,0.));
#13416=DIRECTION('center_axis',(0.,-1.,0.));
#13417=DIRECTION('ref_axis',(0.891006524188368,0.,0.453990499739547));
#13418=DIRECTION('center_axis',(0.,1.,0.));
#13419=DIRECTION('ref_axis',(1.,0.,0.));
#13420=DIRECTION('center_axis',(0.,-1.,0.));
#13421=DIRECTION('ref_axis',(0.951056516295154,0.,0.309016994374948));
#13422=DIRECTION('center_axis',(0.,1.,0.));
#13423=DIRECTION('ref_axis',(1.,0.,0.));
#13424=DIRECTION('center_axis',(0.,1.,0.));
#13425=DIRECTION('ref_axis',(1.,0.,0.));
#13426=DIRECTION('center_axis',(0.,1.,0.));
#13427=DIRECTION('ref_axis',(1.,0.,0.));
#13428=DIRECTION('',(0.,-1.,0.));
#13429=DIRECTION('center_axis',(0.,1.,0.));
#13430=DIRECTION('ref_axis',(1.,0.,0.));
#13431=DIRECTION('center_axis',(0.,1.,0.));
#13432=DIRECTION('ref_axis',(-0.987688340595137,0.,-0.156434465040233));
#13433=DIRECTION('',(0.,-1.,0.));
#13434=DIRECTION('',(0.,1.,0.));
#13435=DIRECTION('center_axis',(0.,1.,0.));
#13436=DIRECTION('ref_axis',(1.,0.,0.));
#13437=DIRECTION('',(0.,-1.,0.));
#13438=DIRECTION('center_axis',(0.,1.,0.));
#13439=DIRECTION('ref_axis',(-0.951056516295153,0.,-0.309016994374949));
#13440=DIRECTION('',(0.,1.,0.));
#13441=DIRECTION('center_axis',(0.,1.,0.));
#13442=DIRECTION('ref_axis',(1.,0.,0.));
#13443=DIRECTION('',(0.,-1.,0.));
#13444=DIRECTION('center_axis',(0.,1.,0.));
#13445=DIRECTION('ref_axis',(-0.891006524188368,0.,-0.453990499739547));
#13446=DIRECTION('',(0.,1.,0.));
#13447=DIRECTION('center_axis',(0.,1.,0.));
#13448=DIRECTION('ref_axis',(1.,0.,0.));
#13449=DIRECTION('',(0.,-1.,0.));
#13450=DIRECTION('center_axis',(0.,1.,0.));
#13451=DIRECTION('ref_axis',(-0.809016994374948,0.,-0.587785252292473));
#13452=DIRECTION('',(0.,1.,0.));
#13453=DIRECTION('center_axis',(0.,1.,0.));
#13454=DIRECTION('ref_axis',(1.,0.,0.));
#13455=DIRECTION('',(0.,-1.,0.));
#13456=DIRECTION('center_axis',(0.,1.,0.));
#13457=DIRECTION('ref_axis',(-0.707106781186547,0.,-0.707106781186548));
#13458=DIRECTION('',(0.,1.,0.));
#13459=DIRECTION('center_axis',(0.,1.,0.));
#13460=DIRECTION('ref_axis',(1.,0.,0.));
#13461=DIRECTION('',(0.,-1.,0.));
#13462=DIRECTION('center_axis',(0.,1.,0.));
#13463=DIRECTION('ref_axis',(-0.587785252292474,0.,-0.809016994374947));
#13464=DIRECTION('',(0.,1.,0.));
#13465=DIRECTION('center_axis',(0.,1.,0.));
#13466=DIRECTION('ref_axis',(1.,0.,0.));
#13467=DIRECTION('',(0.,-1.,0.));
#13468=DIRECTION('center_axis',(0.,1.,0.));
#13469=DIRECTION('ref_axis',(-0.453990499739547,0.,-0.891006524188368));
#13470=DIRECTION('',(0.,1.,0.));
#13471=DIRECTION('center_axis',(0.,1.,0.));
#13472=DIRECTION('ref_axis',(1.,0.,0.));
#13473=DIRECTION('',(0.,-1.,0.));
#13474=DIRECTION('center_axis',(0.,1.,0.));
#13475=DIRECTION('ref_axis',(-0.309016994374948,0.,-0.951056516295153));
#13476=DIRECTION('',(0.,1.,0.));
#13477=DIRECTION('center_axis',(0.,1.,0.));
#13478=DIRECTION('ref_axis',(1.,0.,0.));
#13479=DIRECTION('',(0.,-1.,0.));
#13480=DIRECTION('center_axis',(0.,1.,0.));
#13481=DIRECTION('ref_axis',(-0.156434465040232,0.,-0.987688340595138));
#13482=DIRECTION('',(0.,1.,0.));
#13483=DIRECTION('center_axis',(0.,1.,0.));
#13484=DIRECTION('ref_axis',(1.,0.,0.));
#13485=DIRECTION('',(0.,-1.,0.));
#13486=DIRECTION('center_axis',(0.,1.,0.));
#13487=DIRECTION('ref_axis',(3.06161699786838E-16,0.,-1.));
#13488=DIRECTION('',(0.,1.,0.));
#13489=DIRECTION('center_axis',(0.,1.,0.));
#13490=DIRECTION('ref_axis',(1.,0.,0.));
#13491=DIRECTION('',(0.,-1.,0.));
#13492=DIRECTION('center_axis',(0.,1.,0.));
#13493=DIRECTION('ref_axis',(0.156434465040233,0.,-0.987688340595138));
#13494=DIRECTION('',(0.,1.,0.));
#13495=DIRECTION('center_axis',(0.,1.,0.));
#13496=DIRECTION('ref_axis',(1.,0.,0.));
#13497=DIRECTION('',(0.,-1.,0.));
#13498=DIRECTION('center_axis',(0.,1.,0.));
#13499=DIRECTION('ref_axis',(0.309016994374946,0.,-0.951056516295154));
#13500=DIRECTION('',(0.,1.,0.));
#13501=DIRECTION('center_axis',(0.,1.,0.));
#13502=DIRECTION('ref_axis',(1.,0.,0.));
#13503=DIRECTION('',(0.,-1.,0.));
#13504=DIRECTION('center_axis',(0.,1.,0.));
#13505=DIRECTION('ref_axis',(0.453990499739547,0.,-0.891006524188368));
#13506=DIRECTION('',(0.,1.,0.));
#13507=DIRECTION('center_axis',(0.,1.,0.));
#13508=DIRECTION('ref_axis',(1.,0.,0.));
#13509=DIRECTION('',(0.,-1.,0.));
#13510=DIRECTION('center_axis',(0.,1.,0.));
#13511=DIRECTION('ref_axis',(0.587785252292473,0.,-0.809016994374947));
#13512=DIRECTION('',(0.,1.,0.));
#13513=DIRECTION('center_axis',(0.,1.,0.));
#13514=DIRECTION('ref_axis',(1.,0.,0.));
#13515=DIRECTION('',(0.,-1.,0.));
#13516=DIRECTION('center_axis',(0.,1.,0.));
#13517=DIRECTION('ref_axis',(0.707106781186548,0.,-0.707106781186547));
#13518=DIRECTION('',(0.,1.,0.));
#13519=DIRECTION('center_axis',(0.,1.,0.));
#13520=DIRECTION('ref_axis',(1.,0.,0.));
#13521=DIRECTION('',(0.,-1.,0.));
#13522=DIRECTION('center_axis',(0.,1.,0.));
#13523=DIRECTION('ref_axis',(0.809016994374946,0.,-0.587785252292475));
#13524=DIRECTION('',(0.,1.,0.));
#13525=DIRECTION('center_axis',(0.,1.,0.));
#13526=DIRECTION('ref_axis',(1.,0.,0.));
#13527=DIRECTION('',(0.,-1.,0.));
#13528=DIRECTION('center_axis',(0.,1.,0.));
#13529=DIRECTION('ref_axis',(0.891006524188368,0.,-0.453990499739547));
#13530=DIRECTION('',(0.,1.,0.));
#13531=DIRECTION('center_axis',(0.,1.,0.));
#13532=DIRECTION('ref_axis',(1.,0.,0.));
#13533=DIRECTION('',(0.,-1.,0.));
#13534=DIRECTION('center_axis',(0.,1.,0.));
#13535=DIRECTION('ref_axis',(0.951056516295154,0.,-0.309016994374946));
#13536=DIRECTION('',(0.,1.,0.));
#13537=DIRECTION('center_axis',(0.,1.,0.));
#13538=DIRECTION('ref_axis',(1.,0.,0.));
#13539=DIRECTION('',(0.,-1.,0.));
#13540=DIRECTION('center_axis',(0.,1.,0.));
#13541=DIRECTION('ref_axis',(0.987688340595138,0.,-0.156434465040232));
#13542=DIRECTION('',(0.,1.,0.));
#13543=DIRECTION('center_axis',(0.,1.,0.));
#13544=DIRECTION('ref_axis',(1.,0.,0.));
#13545=DIRECTION('',(0.,-1.,0.));
#13546=DIRECTION('center_axis',(0.,1.,0.));
#13547=DIRECTION('ref_axis',(1.,0.,2.44929359829471E-16));
#13548=DIRECTION('',(0.,1.,0.));
#13549=DIRECTION('center_axis',(0.,1.,0.));
#13550=DIRECTION('ref_axis',(1.,0.,0.));
#13551=DIRECTION('',(0.,-1.,0.));
#13552=DIRECTION('center_axis',(0.,1.,0.));
#13553=DIRECTION('ref_axis',(0.987688340595137,0.,0.156434465040232));
#13554=DIRECTION('',(0.,1.,0.));
#13555=DIRECTION('center_axis',(0.,1.,0.));
#13556=DIRECTION('ref_axis',(1.,0.,0.));
#13557=DIRECTION('',(0.,-1.,0.));
#13558=DIRECTION('center_axis',(0.,1.,0.));
#13559=DIRECTION('ref_axis',(0.951056516295154,0.,0.309016994374946));
#13560=DIRECTION('',(0.,1.,0.));
#13561=DIRECTION('center_axis',(0.,1.,0.));
#13562=DIRECTION('ref_axis',(1.,0.,0.));
#13563=DIRECTION('',(0.,-1.,0.));
#13564=DIRECTION('center_axis',(0.,1.,0.));
#13565=DIRECTION('ref_axis',(0.891006524188368,0.,0.453990499739547));
#13566=DIRECTION('',(0.,1.,0.));
#13567=DIRECTION('center_axis',(0.,1.,0.));
#13568=DIRECTION('ref_axis',(1.,0.,0.));
#13569=DIRECTION('',(0.,-1.,0.));
#13570=DIRECTION('center_axis',(0.,1.,0.));
#13571=DIRECTION('ref_axis',(0.809016994374947,0.,0.587785252292473));
#13572=DIRECTION('',(0.,1.,0.));
#13573=DIRECTION('center_axis',(0.,1.,0.));
#13574=DIRECTION('ref_axis',(1.,0.,0.));
#13575=DIRECTION('',(0.,-1.,0.));
#13576=DIRECTION('center_axis',(0.,1.,0.));
#13577=DIRECTION('ref_axis',(0.707106781186547,0.,0.707106781186548));
#13578=DIRECTION('',(0.,1.,0.));
#13579=DIRECTION('center_axis',(0.,1.,0.));
#13580=DIRECTION('ref_axis',(1.,0.,0.));
#13581=DIRECTION('',(0.,-1.,0.));
#13582=DIRECTION('center_axis',(0.,1.,0.));
#13583=DIRECTION('ref_axis',(0.587785252292475,0.,0.809016994374946));
#13584=DIRECTION('',(0.,1.,0.));
#13585=DIRECTION('center_axis',(0.,1.,0.));
#13586=DIRECTION('ref_axis',(1.,0.,0.));
#13587=DIRECTION('',(0.,-1.,0.));
#13588=DIRECTION('center_axis',(0.,1.,0.));
#13589=DIRECTION('ref_axis',(0.453990499739547,0.,0.891006524188368));
#13590=DIRECTION('',(0.,1.,0.));
#13591=DIRECTION('center_axis',(0.,1.,0.));
#13592=DIRECTION('ref_axis',(1.,0.,0.));
#13593=DIRECTION('',(0.,-1.,0.));
#13594=DIRECTION('center_axis',(0.,1.,0.));
#13595=DIRECTION('ref_axis',(0.309016994374946,0.,0.951056516295154));
#13596=DIRECTION('',(0.,1.,0.));
#13597=DIRECTION('center_axis',(0.,1.,0.));
#13598=DIRECTION('ref_axis',(1.,0.,0.));
#13599=DIRECTION('',(0.,-1.,0.));
#13600=DIRECTION('center_axis',(0.,1.,0.));
#13601=DIRECTION('ref_axis',(0.156434465040232,0.,0.987688340595138));
#13602=DIRECTION('',(0.,1.,0.));
#13603=DIRECTION('center_axis',(0.,1.,0.));
#13604=DIRECTION('ref_axis',(1.,0.,0.));
#13605=DIRECTION('',(0.,-1.,0.));
#13606=DIRECTION('center_axis',(0.,1.,0.));
#13607=DIRECTION('ref_axis',(-1.83697019872103E-16,0.,1.));
#13608=DIRECTION('',(0.,1.,0.));
#13609=DIRECTION('center_axis',(0.,1.,0.));
#13610=DIRECTION('ref_axis',(1.,0.,0.));
#13611=DIRECTION('',(0.,-1.,0.));
#13612=DIRECTION('center_axis',(0.,1.,0.));
#13613=DIRECTION('ref_axis',(-0.156434465040232,0.,0.987688340595138));
#13614=DIRECTION('',(0.,1.,0.));
#13615=DIRECTION('center_axis',(0.,1.,0.));
#13616=DIRECTION('ref_axis',(1.,0.,0.));
#13617=DIRECTION('',(0.,-1.,0.));
#13618=DIRECTION('center_axis',(0.,1.,0.));
#13619=DIRECTION('ref_axis',(-0.309016994374946,0.,0.951056516295154));
#13620=DIRECTION('',(0.,1.,0.));
#13621=DIRECTION('center_axis',(0.,1.,0.));
#13622=DIRECTION('ref_axis',(1.,0.,0.));
#13623=DIRECTION('',(0.,-1.,0.));
#13624=DIRECTION('center_axis',(0.,1.,0.));
#13625=DIRECTION('ref_axis',(-0.453990499739549,0.,0.891006524188367));
#13626=DIRECTION('',(0.,1.,0.));
#13627=DIRECTION('center_axis',(0.,1.,0.));
#13628=DIRECTION('ref_axis',(1.,0.,0.));
#13629=DIRECTION('',(0.,-1.,0.));
#13630=DIRECTION('center_axis',(0.,1.,0.));
#13631=DIRECTION('ref_axis',(-0.587785252292474,0.,0.809016994374947));
#13632=DIRECTION('',(0.,1.,0.));
#13633=DIRECTION('center_axis',(0.,1.,0.));
#13634=DIRECTION('ref_axis',(1.,0.,0.));
#13635=DIRECTION('',(0.,-1.,0.));
#13636=DIRECTION('center_axis',(0.,1.,0.));
#13637=DIRECTION('ref_axis',(-0.707106781186548,0.,0.707106781186547));
#13638=DIRECTION('',(0.,1.,0.));
#13639=DIRECTION('center_axis',(0.,1.,0.));
#13640=DIRECTION('ref_axis',(1.,0.,0.));
#13641=DIRECTION('',(0.,-1.,0.));
#13642=DIRECTION('center_axis',(0.,1.,0.));
#13643=DIRECTION('ref_axis',(-0.809016994374947,0.,0.587785252292474));
#13644=DIRECTION('',(0.,1.,0.));
#13645=DIRECTION('center_axis',(0.,1.,0.));
#13646=DIRECTION('ref_axis',(1.,0.,0.));
#13647=DIRECTION('',(0.,-1.,0.));
#13648=DIRECTION('center_axis',(0.,1.,0.));
#13649=DIRECTION('ref_axis',(-0.891006524188368,0.,0.453990499739547));
#13650=DIRECTION('',(0.,1.,0.));
#13651=DIRECTION('center_axis',(0.,1.,0.));
#13652=DIRECTION('ref_axis',(1.,0.,0.));
#13653=DIRECTION('',(0.,-1.,0.));
#13654=DIRECTION('center_axis',(0.,1.,0.));
#13655=DIRECTION('ref_axis',(-0.951056516295154,0.,0.309016994374948));
#13656=DIRECTION('',(0.,1.,0.));
#13657=DIRECTION('center_axis',(0.,1.,0.));
#13658=DIRECTION('ref_axis',(1.,0.,0.));
#13659=DIRECTION('',(0.,-1.,0.));
#13660=DIRECTION('center_axis',(0.,1.,0.));
#13661=DIRECTION('ref_axis',(-0.987688340595137,0.,0.156434465040233));
#13662=DIRECTION('',(0.,1.,0.));
#13663=DIRECTION('center_axis',(0.,1.,0.));
#13664=DIRECTION('ref_axis',(1.,0.,0.));
#13665=DIRECTION('',(0.,1.,0.));
#13666=DIRECTION('center_axis',(0.,1.,0.));
#13667=DIRECTION('ref_axis',(-1.,0.,-1.22464679914735E-16));
#13668=DIRECTION('',(0.,-1.,0.));
#13669=DIRECTION('center_axis',(0.,1.,0.));
#13670=DIRECTION('ref_axis',(1.,0.,0.));
#16756=CARTESIAN_POINT('',(0.,0.,0.));
#16757=CARTESIAN_POINT('Origin',(0.,-0.5,0.));
#16758=CARTESIAN_POINT('',(-1.,-0.375,-6.12323399573677E-17));
#16759=CARTESIAN_POINT('',(-0.992156741649222,-0.5,0.125));
#16760=CARTESIAN_POINT('Ctrl Pts',(-1.,-0.375,-1.00613961606655E-16));
#16761=CARTESIAN_POINT('Ctrl Pts',(-1.,-0.375,0.0157128711428661));
#16762=CARTESIAN_POINT('Ctrl Pts',(-0.999591823858855,-0.378143583103513,
0.0324619190698278));
#16763=CARTESIAN_POINT('Ctrl Pts',(-0.998116453123232,-0.390905426591754,
0.0632545375991437));
#16764=CARTESIAN_POINT('Ctrl Pts',(-0.997070068816062,-0.400522781657727,
0.0772994769543643));
#16765=CARTESIAN_POINT('Ctrl Pts',(-0.995102104277285,-0.422700615683787,
0.0994773109804239));
#16766=CARTESIAN_POINT('Ctrl Pts',(-0.994052129228928,-0.436745514765346,
0.109094593469654));
#16767=CARTESIAN_POINT('Ctrl Pts',(-0.99256853061881,-0.467537996927464,
0.121856383722779));
#16768=CARTESIAN_POINT('Ctrl Pts',(-0.992156741649222,-0.484286997589363,
0.125));
#16769=CARTESIAN_POINT('Ctrl Pts',(-0.992156741649222,-0.5,0.125));
#16770=CARTESIAN_POINT('',(-1.,-0.625,-6.12323399573677E-17));
#16771=CARTESIAN_POINT('Ctrl Pts',(-1.,-0.625,-4.5102810375397E-17));
#16772=CARTESIAN_POINT('Ctrl Pts',(-1.,-0.625,-0.0157128711428662));
#16773=CARTESIAN_POINT('Ctrl Pts',(-0.999591823858855,-0.621856416896487,
-0.032461919069828));
#16774=CARTESIAN_POINT('Ctrl Pts',(-0.998116453123232,-0.609094573408246,
-0.0632545375991439));
#16775=CARTESIAN_POINT('Ctrl Pts',(-0.997070068816062,-0.599477218342273,
-0.0772994769543645));
#16776=CARTESIAN_POINT('Ctrl Pts',(-0.995102104277285,-0.577299384316213,
-0.0994773109804241));
#16777=CARTESIAN_POINT('Ctrl Pts',(-0.994052129228928,-0.563254485234654,
-0.109094593469655));
#16778=CARTESIAN_POINT('Ctrl Pts',(-0.99256853061881,-0.532462003072536,
-0.121856383722779));
#16779=CARTESIAN_POINT('Ctrl Pts',(-0.992156741649221,-0.515713002410637,
-0.125));
#16780=CARTESIAN_POINT('Ctrl Pts',(-0.992156741649221,-0.484286997589363,
-0.125));
#16781=CARTESIAN_POINT('Ctrl Pts',(-0.99256853061881,-0.467537996927464,
-0.121856383722779));
#16782=CARTESIAN_POINT('Ctrl Pts',(-0.994052129228928,-0.436745514765346,
-0.109094593469655));
#16783=CARTESIAN_POINT('Ctrl Pts',(-0.995102104277285,-0.422700615683787,
-0.0994773109804241));
#16784=CARTESIAN_POINT('Ctrl Pts',(-0.997070068816062,-0.400522781657728,
-0.0772994769543645));
#16785=CARTESIAN_POINT('Ctrl Pts',(-0.998116453123232,-0.390905426591754,
-0.063254537599144));
#16786=CARTESIAN_POINT('Ctrl Pts',(-0.999591823858855,-0.378143583103513,
-0.0324619190698281));
#16787=CARTESIAN_POINT('Ctrl Pts',(-1.,-0.375,-0.0157128711428663));
#16788=CARTESIAN_POINT('Ctrl Pts',(-1.,-0.375,-9.36750677027476E-17));
#16789=CARTESIAN_POINT('Ctrl Pts',(-0.992156741649222,-0.5,0.125));
#16790=CARTESIAN_POINT('Ctrl Pts',(-0.992156741649222,-0.515713002410637,
0.125));
#16791=CARTESIAN_POINT('Ctrl Pts',(-0.99256853061881,-0.532462003072536,
0.121856383722779));
#16792=CARTESIAN_POINT('Ctrl Pts',(-0.994052129228928,-0.563254485234654,
0.109094593469654));
#16793=CARTESIAN_POINT('Ctrl Pts',(-0.995102104277285,-0.577299384316213,
0.0994773109804241));
#16794=CARTESIAN_POINT('Ctrl Pts',(-0.997070068816062,-0.599477218342273,
0.0772994769543644));
#16795=CARTESIAN_POINT('Ctrl Pts',(-0.998116453123232,-0.609094573408246,
0.0632545375991438));
#16796=CARTESIAN_POINT('Ctrl Pts',(-0.999591823858855,-0.621856416896487,
0.0324619190698279));
#16797=CARTESIAN_POINT('Ctrl Pts',(-1.,-0.625,0.0157128711428661));
#16798=CARTESIAN_POINT('Ctrl Pts',(-1.,-0.625,-4.85722573273506E-17));
#16799=CARTESIAN_POINT('',(-0.586834729715275,-0.5,0.125));
#16800=CARTESIAN_POINT('',(-7.65404249467096E-18,-0.5,0.125));
#16801=CARTESIAN_POINT('',(-0.6,-0.625,1.24532753107453E-17));
#16802=CARTESIAN_POINT('Ctrl Pts',(-0.6,-0.625,-4.16333634234434E-17));
#16803=CARTESIAN_POINT('Ctrl Pts',(-0.6,-0.625,0.0157444828659572));
#16804=CARTESIAN_POINT('Ctrl Pts',(-0.599317707212167,-0.621844041497889,
0.0325072544867633));
#16805=CARTESIAN_POINT('Ctrl Pts',(-0.596852269967858,-0.609072857638709,
0.0632914182239686));
#16806=CARTESIAN_POINT('Ctrl Pts',(-0.59510289473619,-0.599460146728784,
0.077316548567853));
#16807=CARTESIAN_POINT('Ctrl Pts',(-0.591804743154611,-0.577315815675743,
0.0994608796208941));
#16808=CARTESIAN_POINT('Ctrl Pts',(-0.590038488226116,-0.563290995658393,
0.109073016834181));
#16809=CARTESIAN_POINT('Ctrl Pts',(-0.587534197873268,-0.532507913768158,
0.121843784097853));
#16810=CARTESIAN_POINT('Ctrl Pts',(-0.586834729715275,-0.515745525063995,
0.125));
#16811=CARTESIAN_POINT('Ctrl Pts',(-0.586834729715275,-0.5,0.125));
#16812=CARTESIAN_POINT('',(-0.586834729715275,-0.5,-0.125));
#16813=CARTESIAN_POINT('Ctrl Pts',(-0.586834729715275,-0.5,-0.125));
#16814=CARTESIAN_POINT('Ctrl Pts',(-0.586834729715275,-0.515745525063995,
-0.125));
#16815=CARTESIAN_POINT('Ctrl Pts',(-0.587534197873268,-0.532507913768158,
-0.121843784097853));
#16816=CARTESIAN_POINT('Ctrl Pts',(-0.590038488226116,-0.563290995658393,
-0.109073016834181));
#16817=CARTESIAN_POINT('Ctrl Pts',(-0.591804743154611,-0.577315815675743,
-0.0994608796208942));
#16818=CARTESIAN_POINT('Ctrl Pts',(-0.59510289473619,-0.599460146728784,
-0.0773165485678531));
#16819=CARTESIAN_POINT('Ctrl Pts',(-0.596852269967858,-0.609072857638709,
-0.0632914182239687));
#16820=CARTESIAN_POINT('Ctrl Pts',(-0.599317707212167,-0.621844041497889,
-0.0325072544867635));
#16821=CARTESIAN_POINT('Ctrl Pts',(-0.6,-0.625,-0.0157444828659573));
#16822=CARTESIAN_POINT('Ctrl Pts',(-0.6,-0.625,-5.20417042793042E-17));
#16823=CARTESIAN_POINT('',(-0.6,-0.375,3.50046804984438E-17));
#16824=CARTESIAN_POINT('Ctrl Pts',(-0.6,-0.375,-3.46944695195361E-18));
#16825=CARTESIAN_POINT('Ctrl Pts',(-0.6,-0.375,-0.0157444828659572));
#16826=CARTESIAN_POINT('Ctrl Pts',(-0.599317707212167,-0.378155958502111,
-0.0325072544867634));
#16827=CARTESIAN_POINT('Ctrl Pts',(-0.596852269967858,-0.390927142361291,
-0.0632914182239686));
#16828=CARTESIAN_POINT('Ctrl Pts',(-0.59510289473619,-0.400539853271216,
-0.077316548567853));
#16829=CARTESIAN_POINT('Ctrl Pts',(-0.591804743154611,-0.422684184324257,
-0.0994608796208942));
#16830=CARTESIAN_POINT('Ctrl Pts',(-0.590038488226116,-0.436709004341607,
-0.109073016834181));
#16831=CARTESIAN_POINT('Ctrl Pts',(-0.587534197873268,-0.467492086231842,
-0.121843784097853));
#16832=CARTESIAN_POINT('Ctrl Pts',(-0.586834729715275,-0.484254474936005,
-0.125));
#16833=CARTESIAN_POINT('Ctrl Pts',(-0.586834729715275,-0.5,-0.125));
#16834=CARTESIAN_POINT('Ctrl Pts',(-0.586834729715275,-0.5,0.125));
#16835=CARTESIAN_POINT('Ctrl Pts',(-0.586834729715275,-0.484254474936005,
0.125));
#16836=CARTESIAN_POINT('Ctrl Pts',(-0.587534197873268,-0.467492086231842,
0.121843784097853));
#16837=CARTESIAN_POINT('Ctrl Pts',(-0.590038488226116,-0.436709004341607,
0.109073016834181));
#16838=CARTESIAN_POINT('Ctrl Pts',(-0.591804743154611,-0.422684184324257,
0.0994608796208941));
#16839=CARTESIAN_POINT('Ctrl Pts',(-0.59510289473619,-0.400539853271216,
0.077316548567853));
#16840=CARTESIAN_POINT('Ctrl Pts',(-0.596852269967858,-0.390927142361291,
0.0632914182239686));
#16841=CARTESIAN_POINT('Ctrl Pts',(-0.599317707212167,-0.378155958502111,
0.0325072544867634));
#16842=CARTESIAN_POINT('Ctrl Pts',(-0.6,-0.375,0.0157444828659572));
#16843=CARTESIAN_POINT('Ctrl Pts',(-0.6,-0.375,-2.42861286636753E-17));
#16844=CARTESIAN_POINT('Origin',(0.,-0.5,0.));
#16845=CARTESIAN_POINT('',(0.586834729715275,-0.5,-0.125));
#16846=CARTESIAN_POINT('',(0.586834729715275,-0.5,0.125));
#16847=CARTESIAN_POINT('Ctrl Pts',(0.586834729715275,-0.5,-0.125));
#16848=CARTESIAN_POINT('Ctrl Pts',(0.586834729715275,-0.484254474936005,
-0.125));
#16849=CARTESIAN_POINT('Ctrl Pts',(0.587534197873268,-0.467492086231842,
-0.121843784097853));
#16850=CARTESIAN_POINT('Ctrl Pts',(0.590038488226116,-0.436709004341607,
-0.109073016834181));
#16851=CARTESIAN_POINT('Ctrl Pts',(0.591804743154611,-0.422684184324257,
-0.0994608796208941));
#16852=CARTESIAN_POINT('Ctrl Pts',(0.59510289473619,-0.400539853271216,
-0.0773165485678529));
#16853=CARTESIAN_POINT('Ctrl Pts',(0.596852269967858,-0.390927142361291,
-0.0632914182239686));
#16854=CARTESIAN_POINT('Ctrl Pts',(0.599317707212167,-0.378155958502111,
-0.0325072544867633));
#16855=CARTESIAN_POINT('Ctrl Pts',(0.6,-0.375,-0.0157444828659572));
#16856=CARTESIAN_POINT('Ctrl Pts',(0.6,-0.375,0.0157444828659573));
#16857=CARTESIAN_POINT('Ctrl Pts',(0.599317707212167,-0.378155958502111,
0.0325072544867635));
#16858=CARTESIAN_POINT('Ctrl Pts',(0.596852269967858,-0.390927142361291,
0.0632914182239687));
#16859=CARTESIAN_POINT('Ctrl Pts',(0.59510289473619,-0.400539853271216,
0.0773165485678531));
#16860=CARTESIAN_POINT('Ctrl Pts',(0.591804743154611,-0.422684184324257,
0.0994608796208942));
#16861=CARTESIAN_POINT('Ctrl Pts',(0.590038488226116,-0.436709004341607,
0.109073016834181));
#16862=CARTESIAN_POINT('Ctrl Pts',(0.587534197873268,-0.467492086231842,
0.121843784097853));
#16863=CARTESIAN_POINT('Ctrl Pts',(0.586834729715275,-0.484254474936005,
0.125));
#16864=CARTESIAN_POINT('Ctrl Pts',(0.586834729715275,-0.5,0.125));
#16865=CARTESIAN_POINT('Ctrl Pts',(0.586834729715275,-0.5,0.125));
#16866=CARTESIAN_POINT('Ctrl Pts',(0.586834729715275,-0.515745525063995,
0.125));
#16867=CARTESIAN_POINT('Ctrl Pts',(0.587534197873268,-0.532507913768158,
0.121843784097853));
#16868=CARTESIAN_POINT('Ctrl Pts',(0.590038488226116,-0.563290995658393,
0.109073016834181));
#16869=CARTESIAN_POINT('Ctrl Pts',(0.591804743154611,-0.577315815675743,
0.0994608796208942));
#16870=CARTESIAN_POINT('Ctrl Pts',(0.59510289473619,-0.599460146728784,
0.077316548567853));
#16871=CARTESIAN_POINT('Ctrl Pts',(0.596852269967858,-0.609072857638709,
0.0632914182239688));
#16872=CARTESIAN_POINT('Ctrl Pts',(0.599317707212167,-0.621844041497889,
0.0325072544867635));
#16873=CARTESIAN_POINT('Ctrl Pts',(0.6,-0.625,0.0157444828659573));
#16874=CARTESIAN_POINT('Ctrl Pts',(0.6,-0.625,-0.0157444828659572));
#16875=CARTESIAN_POINT('Ctrl Pts',(0.599317707212167,-0.621844041497889,
-0.0325072544867633));
#16876=CARTESIAN_POINT('Ctrl Pts',(0.596852269967858,-0.609072857638709,
-0.0632914182239685));
#16877=CARTESIAN_POINT('Ctrl Pts',(0.59510289473619,-0.599460146728784,
-0.077316548567853));
#16878=CARTESIAN_POINT('Ctrl Pts',(0.591804743154611,-0.577315815675743,
-0.0994608796208941));
#16879=CARTESIAN_POINT('Ctrl Pts',(0.590038488226116,-0.563290995658393,
-0.10907301683418));
#16880=CARTESIAN_POINT('Ctrl Pts',(0.587534197873268,-0.532507913768158,
-0.121843784097853));
#16881=CARTESIAN_POINT('Ctrl Pts',(0.586834729715275,-0.515745525063995,
-0.125));
#16882=CARTESIAN_POINT('Ctrl Pts',(0.586834729715275,-0.5,-0.125));
#16883=CARTESIAN_POINT('',(0.992156741649222,-0.5,0.125));
#16884=CARTESIAN_POINT('',(-7.65404249467096E-18,-0.5,0.125));
#16885=CARTESIAN_POINT('',(1.,-0.625,6.12323399573677E-17));
#16886=CARTESIAN_POINT('Ctrl Pts',(1.,-0.625,7.28583859910259E-17));
#16887=CARTESIAN_POINT('Ctrl Pts',(1.,-0.625,0.0157128711428663));
#16888=CARTESIAN_POINT('Ctrl Pts',(0.999591823858855,-0.621856416896487,
0.032461919069828));
#16889=CARTESIAN_POINT('Ctrl Pts',(0.998116453123232,-0.609094573408246,
0.0632545375991439));
#16890=CARTESIAN_POINT('Ctrl Pts',(0.997070068816062,-0.599477218342273,
0.0772994769543645));
#16891=CARTESIAN_POINT('Ctrl Pts',(0.995102104277285,-0.577299384316213,
0.0994773109804242));
#16892=CARTESIAN_POINT('Ctrl Pts',(0.994052129228928,-0.563254485234654,
0.109094593469655));
#16893=CARTESIAN_POINT('Ctrl Pts',(0.99256853061881,-0.532462003072536,
0.121856383722779));
#16894=CARTESIAN_POINT('Ctrl Pts',(0.992156741649222,-0.515713002410637,
0.125));
#16895=CARTESIAN_POINT('Ctrl Pts',(0.992156741649222,-0.5,0.125));
#16896=CARTESIAN_POINT('',(1.,-0.375,6.12323399573677E-17));
#16897=CARTESIAN_POINT('Ctrl Pts',(1.,-0.375,2.08166817117217E-17));
#16898=CARTESIAN_POINT('Ctrl Pts',(1.,-0.375,-0.0157128711428662));
#16899=CARTESIAN_POINT('Ctrl Pts',(0.999591823858855,-0.378143583103513,
-0.032461919069828));
#16900=CARTESIAN_POINT('Ctrl Pts',(0.998116453123232,-0.390905426591754,
-0.0632545375991438));
#16901=CARTESIAN_POINT('Ctrl Pts',(0.997070068816062,-0.400522781657728,
-0.0772994769543644));
#16902=CARTESIAN_POINT('Ctrl Pts',(0.995102104277285,-0.422700615683787,
-0.099477310980424));
#16903=CARTESIAN_POINT('Ctrl Pts',(0.994052129228928,-0.436745514765346,
-0.109094593469654));
#16904=CARTESIAN_POINT('Ctrl Pts',(0.99256853061881,-0.467537996927464,
-0.121856383722779));
#16905=CARTESIAN_POINT('Ctrl Pts',(0.992156741649222,-0.484286997589363,
-0.125));
#16906=CARTESIAN_POINT('Ctrl Pts',(0.992156741649222,-0.515713002410637,
-0.125));
#16907=CARTESIAN_POINT('Ctrl Pts',(0.99256853061881,-0.532462003072536,
-0.121856383722779));
#16908=CARTESIAN_POINT('Ctrl Pts',(0.994052129228928,-0.563254485234654,
-0.109094593469654));
#16909=CARTESIAN_POINT('Ctrl Pts',(0.995102104277285,-0.577299384316213,
-0.099477310980424));
#16910=CARTESIAN_POINT('Ctrl Pts',(0.997070068816062,-0.599477218342273,
-0.0772994769543643));
#16911=CARTESIAN_POINT('Ctrl Pts',(0.998116453123232,-0.609094573408246,
-0.0632545375991438));
#16912=CARTESIAN_POINT('Ctrl Pts',(0.999591823858855,-0.621856416896487,
-0.0324619190698279));
#16913=CARTESIAN_POINT('Ctrl Pts',(1.,-0.625,-0.0157128711428661));
#16914=CARTESIAN_POINT('Ctrl Pts',(1.,-0.625,8.32667268468867E-17));
#16915=CARTESIAN_POINT('Ctrl Pts',(0.992156741649222,-0.5,0.125));
#16916=CARTESIAN_POINT('Ctrl Pts',(0.992156741649222,-0.484286997589363,
0.125));
#16917=CARTESIAN_POINT('Ctrl Pts',(0.99256853061881,-0.467537996927464,
0.121856383722779));
#16918=CARTESIAN_POINT('Ctrl Pts',(0.994052129228928,-0.436745514765346,
0.109094593469654));
#16919=CARTESIAN_POINT('Ctrl Pts',(0.995102104277285,-0.422700615683787,
0.0994773109804241));
#16920=CARTESIAN_POINT('Ctrl Pts',(0.997070068816062,-0.400522781657727,
0.0772994769543644));
#16921=CARTESIAN_POINT('Ctrl Pts',(0.998116453123232,-0.390905426591754,
0.0632545375991438));
#16922=CARTESIAN_POINT('Ctrl Pts',(0.999591823858855,-0.378143583103513,
0.0324619190698279));
#16923=CARTESIAN_POINT('Ctrl Pts',(1.,-0.375,0.0157128711428662));
#16924=CARTESIAN_POINT('Ctrl Pts',(1.,-0.375,2.77555756156289E-17));
#16925=CARTESIAN_POINT('Origin',(0.,-0.1,0.));
#16926=CARTESIAN_POINT('',(-1.,-0.9,1.22464679914735E-16));
#16927=CARTESIAN_POINT('Origin',(0.,-0.9,0.));
#16928=CARTESIAN_POINT('',(-1.,-0.1,-1.22464679914735E-16));
#16929=CARTESIAN_POINT('',(-1.,-0.1,1.22464679914735E-16));
#16930=CARTESIAN_POINT('',(-1.,-0.1,-1.22464679914735E-16));
#16931=CARTESIAN_POINT('Origin',(0.,-0.1,0.));
#16932=CARTESIAN_POINT('',(0.,-0.625,-1.));
#16933=CARTESIAN_POINT('',(0.,-0.375,-1.));
#16934=CARTESIAN_POINT('Ctrl Pts',(-2.08166817117217E-17,-0.625,-1.));
#16935=CARTESIAN_POINT('Ctrl Pts',(0.0157128711428662,-0.625,-1.));
#16936=CARTESIAN_POINT('Ctrl Pts',(0.0324619190698279,-0.621856416896487,
-0.999591823858855));
#16937=CARTESIAN_POINT('Ctrl Pts',(0.0632545375991438,-0.609094573408246,
-0.998116453123232));
#16938=CARTESIAN_POINT('Ctrl Pts',(0.0772994769543644,-0.599477218342273,
-0.997070068816062));
#16939=CARTESIAN_POINT('Ctrl Pts',(0.0994773109804241,-0.577299384316213,
-0.995102104277285));
#16940=CARTESIAN_POINT('Ctrl Pts',(0.109094593469654,-0.563254485234654,
-0.994052129228928));
#16941=CARTESIAN_POINT('Ctrl Pts',(0.121856383722779,-0.532462003072536,
-0.99256853061881));
#16942=CARTESIAN_POINT('Ctrl Pts',(0.125,-0.515713002410637,-0.992156741649221));
#16943=CARTESIAN_POINT('Ctrl Pts',(0.125,-0.484286997589363,-0.992156741649221));
#16944=CARTESIAN_POINT('Ctrl Pts',(0.121856383722779,-0.467537996927464,
-0.99256853061881));
#16945=CARTESIAN_POINT('Ctrl Pts',(0.109094593469654,-0.436745514765346,
-0.994052129228928));
#16946=CARTESIAN_POINT('Ctrl Pts',(0.0994773109804241,-0.422700615683787,
-0.995102104277285));
#16947=CARTESIAN_POINT('Ctrl Pts',(0.0772994769543645,-0.400522781657728,
-0.997070068816062));
#16948=CARTESIAN_POINT('Ctrl Pts',(0.0632545375991439,-0.390905426591754,
-0.998116453123232));
#16949=CARTESIAN_POINT('Ctrl Pts',(0.032461919069828,-0.378143583103513,
-0.999591823858855));
#16950=CARTESIAN_POINT('Ctrl Pts',(0.0157128711428662,-0.375,-1.));
#16951=CARTESIAN_POINT('Ctrl Pts',(3.81639164714898E-17,-0.375,-1.));
#16952=CARTESIAN_POINT('',(-0.125,-0.5,-0.992156741649222));
#16953=CARTESIAN_POINT('Ctrl Pts',(4.5102810375397E-17,-0.375,-1.));
#16954=CARTESIAN_POINT('Ctrl Pts',(-0.0157128711428661,-0.375,-1.));
#16955=CARTESIAN_POINT('Ctrl Pts',(-0.0324619190698279,-0.378143583103513,
-0.999591823858855));
#16956=CARTESIAN_POINT('Ctrl Pts',(-0.0632545375991437,-0.390905426591754,
-0.998116453123232));
#16957=CARTESIAN_POINT('Ctrl Pts',(-0.0772994769543643,-0.400522781657727,
-0.997070068816062));
#16958=CARTESIAN_POINT('Ctrl Pts',(-0.099477310980424,-0.422700615683787,
-0.995102104277285));
#16959=CARTESIAN_POINT('Ctrl Pts',(-0.109094593469654,-0.436745514765346,
-0.994052129228928));
#16960=CARTESIAN_POINT('Ctrl Pts',(-0.121856383722779,-0.467537996927464,
-0.99256853061881));
#16961=CARTESIAN_POINT('Ctrl Pts',(-0.125,-0.484286997589363,-0.992156741649222));
#16962=CARTESIAN_POINT('Ctrl Pts',(-0.125,-0.5,-0.992156741649222));
#16963=CARTESIAN_POINT('Ctrl Pts',(-0.125,-0.5,-0.992156741649222));
#16964=CARTESIAN_POINT('Ctrl Pts',(-0.125,-0.515713002410637,-0.992156741649222));
#16965=CARTESIAN_POINT('Ctrl Pts',(-0.121856383722779,-0.532462003072536,
-0.99256853061881));
#16966=CARTESIAN_POINT('Ctrl Pts',(-0.109094593469654,-0.563254485234654,
-0.994052129228928));
#16967=CARTESIAN_POINT('Ctrl Pts',(-0.0994773109804241,-0.577299384316213,
-0.995102104277285));
#16968=CARTESIAN_POINT('Ctrl Pts',(-0.0772994769543644,-0.599477218342273,
-0.997070068816062));
#16969=CARTESIAN_POINT('Ctrl Pts',(-0.0632545375991439,-0.609094573408246,
-0.998116453123232));
#16970=CARTESIAN_POINT('Ctrl Pts',(-0.032461919069828,-0.621856416896487,
-0.999591823858855));
#16971=CARTESIAN_POINT('Ctrl Pts',(-0.0157128711428662,-0.625,-1.));
#16972=CARTESIAN_POINT('Ctrl Pts',(-1.38777878078145E-17,-0.625,-1.));
#16973=CARTESIAN_POINT('',(0.,-0.375,1.));
#16974=CARTESIAN_POINT('',(0.,-0.625,1.));
#16975=CARTESIAN_POINT('Ctrl Pts',(4.16333634234434E-17,-0.375,1.));
#16976=CARTESIAN_POINT('Ctrl Pts',(0.0157128711428662,-0.375,1.));
#16977=CARTESIAN_POINT('Ctrl Pts',(0.032461919069828,-0.378143583103513,
0.999591823858855));
#16978=CARTESIAN_POINT('Ctrl Pts',(0.0632545375991439,-0.390905426591754,
0.998116453123232));
#16979=CARTESIAN_POINT('Ctrl Pts',(0.0772994769543644,-0.400522781657728,
0.997070068816062));
#16980=CARTESIAN_POINT('Ctrl Pts',(0.0994773109804241,-0.422700615683787,
0.995102104277285));
#16981=CARTESIAN_POINT('Ctrl Pts',(0.109094593469654,-0.436745514765346,
0.994052129228928));
#16982=CARTESIAN_POINT('Ctrl Pts',(0.121856383722779,-0.467537996927464,
0.99256853061881));
#16983=CARTESIAN_POINT('Ctrl Pts',(0.125,-0.484286997589363,0.992156741649222));
#16984=CARTESIAN_POINT('Ctrl Pts',(0.125,-0.515713002410637,0.992156741649222));
#16985=CARTESIAN_POINT('Ctrl Pts',(0.121856383722779,-0.532462003072536,
0.99256853061881));
#16986=CARTESIAN_POINT('Ctrl Pts',(0.109094593469655,-0.563254485234654,
0.994052129228928));
#16987=CARTESIAN_POINT('Ctrl Pts',(0.0994773109804241,-0.577299384316213,
0.995102104277285));
#16988=CARTESIAN_POINT('Ctrl Pts',(0.0772994769543644,-0.599477218342273,
0.997070068816062));
#16989=CARTESIAN_POINT('Ctrl Pts',(0.0632545375991438,-0.609094573408246,
0.998116453123232));
#16990=CARTESIAN_POINT('Ctrl Pts',(0.0324619190698279,-0.621856416896487,
0.999591823858855));
#16991=CARTESIAN_POINT('Ctrl Pts',(0.0157128711428662,-0.625,1.));
#16992=CARTESIAN_POINT('Ctrl Pts',(-1.73472347597681E-17,-0.625,1.));
#16993=CARTESIAN_POINT('',(-0.125,-0.5,0.992156741649222));
#16994=CARTESIAN_POINT('Ctrl Pts',(-1.73472347597681E-17,-0.625,1.));
#16995=CARTESIAN_POINT('Ctrl Pts',(-0.0157128711428662,-0.625,1.));
#16996=CARTESIAN_POINT('Ctrl Pts',(-0.032461919069828,-0.621856416896487,
0.999591823858855));
#16997=CARTESIAN_POINT('Ctrl Pts',(-0.0632545375991439,-0.609094573408246,
0.998116453123232));
#16998=CARTESIAN_POINT('Ctrl Pts',(-0.0772994769543645,-0.599477218342273,
0.997070068816062));
#16999=CARTESIAN_POINT('Ctrl Pts',(-0.0994773109804241,-0.577299384316213,
0.995102104277285));
#17000=CARTESIAN_POINT('Ctrl Pts',(-0.109094593469654,-0.563254485234654,
0.994052129228928));
#17001=CARTESIAN_POINT('Ctrl Pts',(-0.121856383722779,-0.532462003072536,
0.99256853061881));
#17002=CARTESIAN_POINT('Ctrl Pts',(-0.125,-0.515713002410637,0.992156741649222));
#17003=CARTESIAN_POINT('Ctrl Pts',(-0.125,-0.5,0.992156741649222));
#17004=CARTESIAN_POINT('Ctrl Pts',(-0.125,-0.5,0.992156741649222));
#17005=CARTESIAN_POINT('Ctrl Pts',(-0.125,-0.484286997589363,0.992156741649222));
#17006=CARTESIAN_POINT('Ctrl Pts',(-0.121856383722779,-0.467537996927464,
0.99256853061881));
#17007=CARTESIAN_POINT('Ctrl Pts',(-0.109094593469654,-0.436745514765346,
0.994052129228928));
#17008=CARTESIAN_POINT('Ctrl Pts',(-0.099477310980424,-0.422700615683787,
0.995102104277285));
#17009=CARTESIAN_POINT('Ctrl Pts',(-0.0772994769543643,-0.400522781657727,
0.997070068816062));
#17010=CARTESIAN_POINT('Ctrl Pts',(-0.0632545375991438,-0.390905426591754,
0.998116453123232));
#17011=CARTESIAN_POINT('Ctrl Pts',(-0.0324619190698279,-0.378143583103513,
0.999591823858855));
#17012=CARTESIAN_POINT('Ctrl Pts',(-0.0157128711428661,-0.375,1.));
#17013=CARTESIAN_POINT('Ctrl Pts',(4.5102810375397E-17,-0.375,1.));
#17014=CARTESIAN_POINT('Origin',(0.,-0.5,0.));
#17015=CARTESIAN_POINT('',(-0.125,-0.5,-0.586834729715275));
#17016=CARTESIAN_POINT('',(-0.125,-0.5,0.));
#17017=CARTESIAN_POINT('',(0.125,-0.5,-0.586834729715275));
#17018=CARTESIAN_POINT('Ctrl Pts',(0.125,-0.5,-0.586834729715275));
#17019=CARTESIAN_POINT('Ctrl Pts',(0.125,-0.515745525063995,-0.586834729715275));
#17020=CARTESIAN_POINT('Ctrl Pts',(0.121843784097853,-0.532507913768158,
-0.587534197873268));
#17021=CARTESIAN_POINT('Ctrl Pts',(0.109073016834181,-0.563290995658393,
-0.590038488226116));
#17022=CARTESIAN_POINT('Ctrl Pts',(0.0994608796208942,-0.577315815675743,
-0.591804743154611));
#17023=CARTESIAN_POINT('Ctrl Pts',(0.077316548567853,-0.599460146728784,
-0.59510289473619));
#17024=CARTESIAN_POINT('Ctrl Pts',(0.0632914182239686,-0.609072857638709,
-0.596852269967858));
#17025=CARTESIAN_POINT('Ctrl Pts',(0.0325072544867633,-0.621844041497889,
-0.599317707212167));
#17026=CARTESIAN_POINT('Ctrl Pts',(0.0157444828659573,-0.625,-0.6));
#17027=CARTESIAN_POINT('Ctrl Pts',(-0.0157444828659572,-0.625,-0.6));
#17028=CARTESIAN_POINT('Ctrl Pts',(-0.0325072544867633,-0.621844041497889,
-0.599317707212167));
#17029=CARTESIAN_POINT('Ctrl Pts',(-0.0632914182239686,-0.609072857638709,
-0.596852269967858));
#17030=CARTESIAN_POINT('Ctrl Pts',(-0.077316548567853,-0.599460146728784,
-0.59510289473619));
#17031=CARTESIAN_POINT('Ctrl Pts',(-0.0994608796208941,-0.577315815675743,
-0.591804743154611));
#17032=CARTESIAN_POINT('Ctrl Pts',(-0.109073016834181,-0.563290995658393,
-0.590038488226116));
#17033=CARTESIAN_POINT('Ctrl Pts',(-0.121843784097853,-0.532507913768158,
-0.587534197873268));
#17034=CARTESIAN_POINT('Ctrl Pts',(-0.125,-0.515745525063995,-0.586834729715275));
#17035=CARTESIAN_POINT('Ctrl Pts',(-0.125,-0.5,-0.586834729715275));
#17036=CARTESIAN_POINT('Ctrl Pts',(-0.125,-0.5,-0.586834729715275));
#17037=CARTESIAN_POINT('Ctrl Pts',(-0.125,-0.484254474936005,-0.586834729715275));
#17038=CARTESIAN_POINT('Ctrl Pts',(-0.121843784097853,-0.467492086231842,
-0.587534197873268));
#17039=CARTESIAN_POINT('Ctrl Pts',(-0.109073016834181,-0.436709004341607,
-0.590038488226116));
#17040=CARTESIAN_POINT('Ctrl Pts',(-0.0994608796208942,-0.422684184324257,
-0.591804743154611));
#17041=CARTESIAN_POINT('Ctrl Pts',(-0.077316548567853,-0.400539853271216,
-0.59510289473619));
#17042=CARTESIAN_POINT('Ctrl Pts',(-0.0632914182239687,-0.39092714236129,
-0.596852269967858));
#17043=CARTESIAN_POINT('Ctrl Pts',(-0.0325072544867634,-0.378155958502111,
-0.599317707212167));
#17044=CARTESIAN_POINT('Ctrl Pts',(-0.0157444828659573,-0.375,-0.6));
#17045=CARTESIAN_POINT('Ctrl Pts',(0.0157444828659572,-0.375,-0.6));
#17046=CARTESIAN_POINT('Ctrl Pts',(0.0325072544867634,-0.378155958502111,
-0.599317707212167));
#17047=CARTESIAN_POINT('Ctrl Pts',(0.0632914182239686,-0.390927142361291,
-0.596852269967858));
#17048=CARTESIAN_POINT('Ctrl Pts',(0.077316548567853,-0.400539853271216,
-0.59510289473619));
#17049=CARTESIAN_POINT('Ctrl Pts',(0.0994608796208941,-0.422684184324257,
-0.591804743154611));
#17050=CARTESIAN_POINT('Ctrl Pts',(0.109073016834181,-0.436709004341607,
-0.590038488226116));
#17051=CARTESIAN_POINT('Ctrl Pts',(0.121843784097853,-0.467492086231842,
-0.587534197873268));
#17052=CARTESIAN_POINT('Ctrl Pts',(0.125,-0.484254474936005,-0.586834729715275));
#17053=CARTESIAN_POINT('Ctrl Pts',(0.125,-0.5,-0.586834729715275));
#17054=CARTESIAN_POINT('Origin',(0.,-0.5,0.));
#17055=CARTESIAN_POINT('',(0.125,-0.5,0.586834729715275));
#17056=CARTESIAN_POINT('',(-0.125,-0.5,0.586834729715275));
#17057=CARTESIAN_POINT('Ctrl Pts',(0.125,-0.5,0.586834729715275));
#17058=CARTESIAN_POINT('Ctrl Pts',(0.125,-0.484254474936005,0.586834729715275));
#17059=CARTESIAN_POINT('Ctrl Pts',(0.121843784097853,-0.467492086231842,
0.587534197873268));
#17060=CARTESIAN_POINT('Ctrl Pts',(0.109073016834181,-0.436709004341607,
0.590038488226116));
#17061=CARTESIAN_POINT('Ctrl Pts',(0.0994608796208941,-0.422684184324257,
0.591804743154611));
#17062=CARTESIAN_POINT('Ctrl Pts',(0.077316548567853,-0.400539853271216,
0.59510289473619));
#17063=CARTESIAN_POINT('Ctrl Pts',(0.0632914182239686,-0.390927142361291,
0.596852269967858));
#17064=CARTESIAN_POINT('Ctrl Pts',(0.0325072544867634,-0.378155958502111,
0.599317707212167));
#17065=CARTESIAN_POINT('Ctrl Pts',(0.0157444828659572,-0.375,0.6));
#17066=CARTESIAN_POINT('Ctrl Pts',(-0.0157444828659573,-0.375,0.6));
#17067=CARTESIAN_POINT('Ctrl Pts',(-0.0325072544867634,-0.378155958502111,
0.599317707212167));
#17068=CARTESIAN_POINT('Ctrl Pts',(-0.0632914182239687,-0.390927142361291,
0.596852269967858));
#17069=CARTESIAN_POINT('Ctrl Pts',(-0.077316548567853,-0.400539853271216,
0.59510289473619));
#17070=CARTESIAN_POINT('Ctrl Pts',(-0.0994608796208942,-0.422684184324257,
0.591804743154611));
#17071=CARTESIAN_POINT('Ctrl Pts',(-0.109073016834181,-0.436709004341607,
0.590038488226116));
#17072=CARTESIAN_POINT('Ctrl Pts',(-0.121843784097853,-0.467492086231842,
0.587534197873268));
#17073=CARTESIAN_POINT('Ctrl Pts',(-0.125,-0.484254474936005,0.586834729715275));
#17074=CARTESIAN_POINT('Ctrl Pts',(-0.125,-0.5,0.586834729715275));
#17075=CARTESIAN_POINT('Ctrl Pts',(-0.125,-0.5,0.586834729715275));
#17076=CARTESIAN_POINT('Ctrl Pts',(-0.125,-0.515745525063995,0.586834729715275));
#17077=CARTESIAN_POINT('Ctrl Pts',(-0.121843784097853,-0.532507913768158,
0.587534197873268));
#17078=CARTESIAN_POINT('Ctrl Pts',(-0.109073016834181,-0.563290995658393,
0.590038488226116));
#17079=CARTESIAN_POINT('Ctrl Pts',(-0.0994608796208941,-0.577315815675743,
0.591804743154611));
#17080=CARTESIAN_POINT('Ctrl Pts',(-0.077316548567853,-0.599460146728784,
0.59510289473619));
#17081=CARTESIAN_POINT('Ctrl Pts',(-0.0632914182239687,-0.609072857638709,
0.596852269967858));
#17082=CARTESIAN_POINT('Ctrl Pts',(-0.0325072544867635,-0.621844041497889,
0.599317707212167));
#17083=CARTESIAN_POINT('Ctrl Pts',(-0.0157444828659572,-0.625,0.6));
#17084=CARTESIAN_POINT('Ctrl Pts',(0.0157444828659572,-0.625,0.6));
#17085=CARTESIAN_POINT('Ctrl Pts',(0.0325072544867633,-0.621844041497889,
0.599317707212167));
#17086=CARTESIAN_POINT('Ctrl Pts',(0.0632914182239686,-0.609072857638709,
0.596852269967858));
#17087=CARTESIAN_POINT('Ctrl Pts',(0.077316548567853,-0.599460146728784,
0.59510289473619));
#17088=CARTESIAN_POINT('Ctrl Pts',(0.0994608796208942,-0.577315815675743,
0.591804743154611));
#17089=CARTESIAN_POINT('Ctrl Pts',(0.109073016834181,-0.563290995658393,
0.590038488226116));
#17090=CARTESIAN_POINT('Ctrl Pts',(0.121843784097853,-0.532507913768158,
0.587534197873268));
#17091=CARTESIAN_POINT('Ctrl Pts',(0.125,-0.515745525063995,0.586834729715275));
#17092=CARTESIAN_POINT('Ctrl Pts',(0.125,-0.5,0.586834729715275));
#17093=CARTESIAN_POINT('',(-0.125,-0.5,0.));
#17094=CARTESIAN_POINT('Origin',(0.,0.,0.));
#17095=CARTESIAN_POINT('',(-0.6,-0.9,7.34788079488412E-17));
#17096=CARTESIAN_POINT('Origin',(0.,-0.9,0.));
#17097=CARTESIAN_POINT('',(-0.6,0.,7.34788079488412E-17));
#17098=CARTESIAN_POINT('',(-0.6,0.85,-7.34788079488412E-17));
#17099=CARTESIAN_POINT('',(-0.6,0.,7.34788079488412E-17));
#17100=CARTESIAN_POINT('Origin',(0.,0.85,0.));
#17101=CARTESIAN_POINT('Origin',(0.,-0.9,0.));
#17102=CARTESIAN_POINT('Origin',(0.,0.,0.));
#17103=CARTESIAN_POINT('',(-1.4,0.,1.71450551880629E-16));
#17104=CARTESIAN_POINT('Origin',(0.,0.,0.));
#17105=CARTESIAN_POINT('',(1.23958209161204,0.,0.143317017690053));
#17106=CARTESIAN_POINT('',(1.22320001975977,0.,0.246749348660852));
#17107=CARTESIAN_POINT('Origin',(1.21321664662686,0.,0.192154639568406));
#17108=CARTESIAN_POINT('',(1.20190105810224,0.,0.335465908756113));
#17109=CARTESIAN_POINT('Origin',(0.,0.,0.));
#17110=CARTESIAN_POINT('',(1.16954029537568,0.,0.435062095450087));
#17111=CARTESIAN_POINT('Origin',(1.1682203282434,0.,0.379577794185952));
#17112=CARTESIAN_POINT('',(1.13462523166105,0.,0.519354515801077));
#17113=CARTESIAN_POINT('Origin',(0.,0.,0.));
#17114=CARTESIAN_POINT('',(1.08708260743774,0.,0.612662169561029));
#17115=CARTESIAN_POINT('Origin',(1.0944585482776,0.,0.557654483764164));
#17116=CARTESIAN_POINT('',(1.0394111664111,0.,0.690454891028201));
#17117=CARTESIAN_POINT('Origin',(0.,0.,0.));
#17118=CARTESIAN_POINT('',(0.977857337884349,0.,0.775176467748211));
#17119=CARTESIAN_POINT('Origin',(0.993747566553533,0.,0.72199986920298));
#17120=CARTESIAN_POINT('',(0.918603348636233,0.,0.844553975349804));
#17121=CARTESIAN_POINT('Origin',(0.,0.,0.));
#17122=CARTESIAN_POINT('',(0.844553975349804,0.,0.918603348636233));
#17123=CARTESIAN_POINT('Origin',(0.86856722168183,0.,0.86856722168183));
#17124=CARTESIAN_POINT('',(0.775176467748211,0.,0.977857337884349));
#17125=CARTESIAN_POINT('Origin',(0.,0.,0.));
#17126=CARTESIAN_POINT('',(0.690454891028201,0.,1.0394111664111));
#17127=CARTESIAN_POINT('Origin',(0.721999869202979,0.,0.993747566553533));
#17128=CARTESIAN_POINT('',(0.612662169561028,0.,1.08708260743774));
#17129=CARTESIAN_POINT('Origin',(0.,0.,0.));
#17130=CARTESIAN_POINT('',(0.519354515801077,0.,1.13462523166105));
#17131=CARTESIAN_POINT('Origin',(0.557654483764164,0.,1.0944585482776));
#17132=CARTESIAN_POINT('',(0.435062095450087,0.,1.16954029537568));
#17133=CARTESIAN_POINT('Origin',(0.,0.,0.));
#17134=CARTESIAN_POINT('',(0.335465908756113,0.,1.20190105810224));
#17135=CARTESIAN_POINT('Origin',(0.379577794185951,0.,1.1682203282434));
#17136=CARTESIAN_POINT('',(0.246749348660851,0.,1.22320001975977));
#17137=CARTESIAN_POINT('Origin',(0.,0.,0.));
#17138=CARTESIAN_POINT('',(0.143317017690053,0.,1.23958209161204));
#17139=CARTESIAN_POINT('Origin',(0.192154639568406,0.,1.21321664662686));
#17140=CARTESIAN_POINT('',(0.0523608139934478,0.,1.24674050008925));
#17141=CARTESIAN_POINT('Origin',(0.,0.,0.));
#17142=CARTESIAN_POINT('',(-0.0523608139934483,0.,1.24674050008925));
#17143=CARTESIAN_POINT('Origin',(-2.25642313758905E-16,0.,1.22833954473516));
#17144=CARTESIAN_POINT('',(-0.143317017690053,0.,1.23958209161204));
#17145=CARTESIAN_POINT('Origin',(0.,0.,0.));
#17146=CARTESIAN_POINT('',(-0.246749348660852,0.,1.22320001975977));
#17147=CARTESIAN_POINT('Origin',(-0.192154639568406,0.,1.21321664662686));
#17148=CARTESIAN_POINT('',(-0.335465908756113,0.,1.20190105810224));
#17149=CARTESIAN_POINT('Origin',(0.,0.,0.));
#17150=CARTESIAN_POINT('',(-0.435062095450087,0.,1.16954029537568));
#17151=CARTESIAN_POINT('Origin',(-0.379577794185951,0.,1.1682203282434));
#17152=CARTESIAN_POINT('',(-0.519354515801077,0.,1.13462523166105));
#17153=CARTESIAN_POINT('Origin',(0.,0.,0.));
#17154=CARTESIAN_POINT('',(-0.612662169561029,0.,1.08708260743774));
#17155=CARTESIAN_POINT('Origin',(-0.557654483764164,0.,1.0944585482776));
#17156=CARTESIAN_POINT('',(-0.690454891028201,0.,1.0394111664111));
#17157=CARTESIAN_POINT('Origin',(0.,0.,0.));
#17158=CARTESIAN_POINT('',(-0.775176467748211,0.,0.977857337884349));
#17159=CARTESIAN_POINT('Origin',(-0.721999869202979,0.,0.993747566553533));
#17160=CARTESIAN_POINT('',(-0.844553975349804,0.,0.918603348636233));
#17161=CARTESIAN_POINT('Origin',(0.,0.,0.));
#17162=CARTESIAN_POINT('',(-0.918603348636233,0.,0.844553975349804));
#17163=CARTESIAN_POINT('Origin',(-0.86856722168183,0.,0.86856722168183));
#17164=CARTESIAN_POINT('',(-0.977857337884348,0.,0.775176467748211));
#17165=CARTESIAN_POINT('Origin',(0.,0.,0.));
#17166=CARTESIAN_POINT('',(-1.0394111664111,0.,0.690454891028201));
#17167=CARTESIAN_POINT('Origin',(-0.993747566553533,0.,0.721999869202979));
#17168=CARTESIAN_POINT('',(-1.08708260743774,0.,0.612662169561028));
#17169=CARTESIAN_POINT('Origin',(0.,0.,0.));
#17170=CARTESIAN_POINT('',(-1.13462523166105,0.,0.519354515801077));
#17171=CARTESIAN_POINT('Origin',(-1.0944585482776,0.,0.557654483764164));
#17172=CARTESIAN_POINT('',(-1.16954029537568,0.,0.435062095450087));
#17173=CARTESIAN_POINT('Origin',(0.,0.,0.));
#17174=CARTESIAN_POINT('',(-1.20190105810224,0.,0.335465908756113));
#17175=CARTESIAN_POINT('Origin',(-1.1682203282434,0.,0.379577794185951));
#17176=CARTESIAN_POINT('',(-1.22320001975977,0.,0.246749348660851));
#17177=CARTESIAN_POINT('Origin',(0.,0.,0.));
#17178=CARTESIAN_POINT('',(-1.23958209161204,0.,0.143317017690053));
#17179=CARTESIAN_POINT('Origin',(-1.21321664662686,0.,0.192154639568406));
#17180=CARTESIAN_POINT('',(-1.24674050008925,0.,0.0523608139934479));
#17181=CARTESIAN_POINT('Origin',(0.,0.,0.));
#17182=CARTESIAN_POINT('',(-1.24674050008925,0.,-0.0523608139934482));
#17183=CARTESIAN_POINT('Origin',(-1.22833954473516,0.,-1.50428209172603E-16));
#17184=CARTESIAN_POINT('',(-1.23958209161204,0.,-0.143317017690053));
#17185=CARTESIAN_POINT('Origin',(0.,0.,0.));
#17186=CARTESIAN_POINT('',(-1.22320001975977,0.,-0.246749348660852));
#17187=CARTESIAN_POINT('Origin',(-1.21321664662686,0.,-0.192154639568406));
#17188=CARTESIAN_POINT('',(-1.20190105810224,0.,-0.335465908756113));
#17189=CARTESIAN_POINT('Origin',(0.,0.,0.));
#17190=CARTESIAN_POINT('',(-1.16954029537568,0.,-0.435062095450087));
#17191=CARTESIAN_POINT('Origin',(-1.1682203282434,0.,-0.379577794185951));
#17192=CARTESIAN_POINT('',(-1.13462523166105,0.,-0.519354515801077));
#17193=CARTESIAN_POINT('Origin',(0.,0.,0.));
#17194=CARTESIAN_POINT('',(-1.08708260743774,0.,-0.612662169561029));
#17195=CARTESIAN_POINT('Origin',(-1.0944585482776,0.,-0.557654483764164));
#17196=CARTESIAN_POINT('',(-1.0394111664111,0.,-0.690454891028201));
#17197=CARTESIAN_POINT('Origin',(0.,0.,0.));
#17198=CARTESIAN_POINT('',(-0.977857337884349,0.,-0.775176467748211));
#17199=CARTESIAN_POINT('Origin',(-0.993747566553533,0.,-0.721999869202979));
#17200=CARTESIAN_POINT('',(-0.918603348636233,0.,-0.844553975349804));
#17201=CARTESIAN_POINT('Origin',(0.,0.,0.));
#17202=CARTESIAN_POINT('',(-0.844553975349804,0.,-0.918603348636233));
#17203=CARTESIAN_POINT('Origin',(-0.86856722168183,0.,-0.86856722168183));
#17204=CARTESIAN_POINT('',(-0.775176467748211,0.,-0.977857337884348));
#17205=CARTESIAN_POINT('Origin',(0.,0.,0.));
#17206=CARTESIAN_POINT('',(-0.690454891028201,0.,-1.0394111664111));
#17207=CARTESIAN_POINT('Origin',(-0.721999869202979,0.,-0.993747566553533));
#17208=CARTESIAN_POINT('',(-0.612662169561028,0.,-1.08708260743774));
#17209=CARTESIAN_POINT('Origin',(0.,0.,0.));
#17210=CARTESIAN_POINT('',(-0.519354515801077,0.,-1.13462523166105));
#17211=CARTESIAN_POINT('Origin',(-0.557654483764164,0.,-1.0944585482776));
#17212=CARTESIAN_POINT('',(-0.435062095450087,0.,-1.16954029537568));
#17213=CARTESIAN_POINT('Origin',(0.,0.,0.));
#17214=CARTESIAN_POINT('',(-0.335465908756113,0.,-1.20190105810224));
#17215=CARTESIAN_POINT('Origin',(-0.379577794185951,0.,-1.1682203282434));
#17216=CARTESIAN_POINT('',(-0.246749348660852,0.,-1.22320001975977));
#17217=CARTESIAN_POINT('Origin',(0.,0.,0.));
#17218=CARTESIAN_POINT('',(-0.143317017690053,0.,-1.23958209161204));
#17219=CARTESIAN_POINT('Origin',(-0.192154639568406,0.,-1.21321664662686));
#17220=CARTESIAN_POINT('',(-0.0523608139934479,0.,-1.24674050008925));
#17221=CARTESIAN_POINT('Origin',(0.,0.,0.));
#17222=CARTESIAN_POINT('',(0.0523608139934481,0.,-1.24674050008925));
#17223=CARTESIAN_POINT('Origin',(7.52141045863017E-17,0.,-1.22833954473516));
#17224=CARTESIAN_POINT('',(0.143317017690053,0.,-1.23958209161204));
#17225=CARTESIAN_POINT('Origin',(0.,0.,0.));
#17226=CARTESIAN_POINT('',(0.246749348660852,0.,-1.22320001975977));
#17227=CARTESIAN_POINT('Origin',(0.192154639568406,0.,-1.21321664662686));
#17228=CARTESIAN_POINT('',(0.335465908756113,0.,-1.20190105810224));
#17229=CARTESIAN_POINT('Origin',(0.,0.,0.));
#17230=CARTESIAN_POINT('',(0.435062095450087,0.,-1.16954029537568));
#17231=CARTESIAN_POINT('Origin',(0.379577794185951,0.,-1.1682203282434));
#17232=CARTESIAN_POINT('',(0.519354515801077,0.,-1.13462523166105));
#17233=CARTESIAN_POINT('Origin',(0.,0.,0.));
#17234=CARTESIAN_POINT('',(0.612662169561028,0.,-1.08708260743774));
#17235=CARTESIAN_POINT('Origin',(0.557654483764164,0.,-1.0944585482776));
#17236=CARTESIAN_POINT('',(0.690454891028201,0.,-1.0394111664111));
#17237=CARTESIAN_POINT('Origin',(0.,0.,0.));
#17238=CARTESIAN_POINT('',(0.775176467748211,0.,-0.977857337884349));
#17239=CARTESIAN_POINT('Origin',(0.721999869202979,0.,-0.993747566553533));
#17240=CARTESIAN_POINT('',(0.844553975349804,0.,-0.918603348636233));
#17241=CARTESIAN_POINT('Origin',(0.,0.,0.));
#17242=CARTESIAN_POINT('',(0.918603348636233,0.,-0.844553975349804));
#17243=CARTESIAN_POINT('Origin',(0.86856722168183,0.,-0.86856722168183));
#17244=CARTESIAN_POINT('',(0.977857337884349,0.,-0.775176467748211));
#17245=CARTESIAN_POINT('Origin',(0.,0.,0.));
#17246=CARTESIAN_POINT('',(1.0394111664111,0.,-0.690454891028201));
#17247=CARTESIAN_POINT('Origin',(0.993747566553533,0.,-0.721999869202979));
#17248=CARTESIAN_POINT('',(1.08708260743774,0.,-0.612662169561028));
#17249=CARTESIAN_POINT('Origin',(0.,0.,0.));
#17250=CARTESIAN_POINT('',(1.13462523166105,0.,-0.519354515801077));
#17251=CARTESIAN_POINT('Origin',(1.0944585482776,0.,-0.557654483764164));
#17252=CARTESIAN_POINT('',(1.16954029537568,0.,-0.43506209545009));
#17253=CARTESIAN_POINT('Origin',(0.,0.,0.));
#17254=CARTESIAN_POINT('',(1.20190105810224,0.,-0.33546590875611));
#17255=CARTESIAN_POINT('Origin',(1.1682203282434,0.,-0.379577794185951));
#17256=CARTESIAN_POINT('',(1.22320001975977,0.,-0.246749348660852));
#17257=CARTESIAN_POINT('Origin',(0.,0.,0.));
#17258=CARTESIAN_POINT('',(1.23958209161204,0.,-0.143317017690053));
#17259=CARTESIAN_POINT('Origin',(1.21321664662686,0.,-0.192154639568406));
#17260=CARTESIAN_POINT('',(1.24674050008925,0.,-0.052360813993451));
#17261=CARTESIAN_POINT('Origin',(0.,0.,0.));
#17262=CARTESIAN_POINT('',(1.24674050008925,0.,0.052360813993451));
#17263=CARTESIAN_POINT('Origin',(1.22833954473516,0.,0.));
#17264=CARTESIAN_POINT('Origin',(0.,0.,0.));
#17265=CARTESIAN_POINT('Origin',(0.,0.,0.));
#17266=CARTESIAN_POINT('',(-1.4,-0.1,1.71450551880629E-16));
#17267=CARTESIAN_POINT('Origin',(0.,-0.1,0.));
#17268=CARTESIAN_POINT('',(-1.4,0.,-1.71450551880629E-16));
#17269=CARTESIAN_POINT('Origin',(0.,-0.1,0.));
#17270=CARTESIAN_POINT('Origin',(0.,0.75,0.));
#17271=CARTESIAN_POINT('',(-1.4,0.75,1.71450551880629E-16));
#17272=CARTESIAN_POINT('Origin',(0.,0.75,0.));
#17273=CARTESIAN_POINT('',(1.22320001975977,0.75,0.246749348660852));
#17274=CARTESIAN_POINT('',(1.23958209161204,0.75,0.143317017690053));
#17275=CARTESIAN_POINT('Origin',(1.21321664662686,0.75,0.192154639568406));
#17276=CARTESIAN_POINT('',(1.24674050008925,0.75,0.052360813993448));
#17277=CARTESIAN_POINT('Origin',(0.,0.75,0.));
#17278=CARTESIAN_POINT('',(1.24674050008925,0.75,-0.052360813993448));
#17279=CARTESIAN_POINT('Origin',(1.22833954473516,0.75,0.));
#17280=CARTESIAN_POINT('',(1.23958209161204,0.75,-0.143317017690053));
#17281=CARTESIAN_POINT('Origin',(0.,0.75,0.));
#17282=CARTESIAN_POINT('',(1.22320001975977,0.75,-0.246749348660852));
#17283=CARTESIAN_POINT('Origin',(1.21321664662686,0.75,-0.192154639568406));
#17284=CARTESIAN_POINT('',(1.20190105810224,0.75,-0.335465908756113));
#17285=CARTESIAN_POINT('Origin',(0.,0.75,0.));
#17286=CARTESIAN_POINT('',(1.16954029537568,0.75,-0.435062095450087));
#17287=CARTESIAN_POINT('Origin',(1.1682203282434,0.75,-0.379577794185951));
#17288=CARTESIAN_POINT('',(1.13462523166105,0.75,-0.519354515801077));
#17289=CARTESIAN_POINT('Origin',(0.,0.75,0.));
#17290=CARTESIAN_POINT('',(1.08708260743774,0.75,-0.612662169561028));
#17291=CARTESIAN_POINT('Origin',(1.0944585482776,0.75,-0.557654483764164));
#17292=CARTESIAN_POINT('',(1.0394111664111,0.75,-0.690454891028201));
#17293=CARTESIAN_POINT('Origin',(0.,0.75,0.));
#17294=CARTESIAN_POINT('',(0.977857337884349,0.75,-0.775176467748211));
#17295=CARTESIAN_POINT('Origin',(0.993747566553533,0.75,-0.721999869202979));
#17296=CARTESIAN_POINT('',(0.918603348636233,0.75,-0.844553975349804));
#17297=CARTESIAN_POINT('Origin',(0.,0.75,0.));
#17298=CARTESIAN_POINT('',(0.844553975349804,0.75,-0.918603348636233));
#17299=CARTESIAN_POINT('Origin',(0.86856722168183,0.75,-0.86856722168183));
#17300=CARTESIAN_POINT('',(0.775176467748211,0.75,-0.977857337884349));
#17301=CARTESIAN_POINT('Origin',(0.,0.75,0.));
#17302=CARTESIAN_POINT('',(0.690454891028201,0.75,-1.0394111664111));
#17303=CARTESIAN_POINT('Origin',(0.721999869202979,0.75,-0.993747566553533));
#17304=CARTESIAN_POINT('',(0.612662169561028,0.75,-1.08708260743774));
#17305=CARTESIAN_POINT('Origin',(0.,0.75,0.));
#17306=CARTESIAN_POINT('',(0.519354515801077,0.75,-1.13462523166105));
#17307=CARTESIAN_POINT('Origin',(0.557654483764164,0.75,-1.0944585482776));
#17308=CARTESIAN_POINT('',(0.435062095450087,0.75,-1.16954029537568));
#17309=CARTESIAN_POINT('Origin',(0.,0.75,0.));
#17310=CARTESIAN_POINT('',(0.335465908756113,0.75,-1.20190105810224));
#17311=CARTESIAN_POINT('Origin',(0.379577794185951,0.75,-1.1682203282434));
#17312=CARTESIAN_POINT('',(0.246749348660852,0.75,-1.22320001975977));
#17313=CARTESIAN_POINT('Origin',(0.,0.75,0.));
#17314=CARTESIAN_POINT('',(0.143317017690053,0.75,-1.23958209161204));
#17315=CARTESIAN_POINT('Origin',(0.192154639568406,0.75,-1.21321664662686));
#17316=CARTESIAN_POINT('',(0.0523608139934481,0.75,-1.24674050008925));
#17317=CARTESIAN_POINT('Origin',(0.,0.75,0.));
#17318=CARTESIAN_POINT('',(-0.0523608139934479,0.75,-1.24674050008925));
#17319=CARTESIAN_POINT('Origin',(7.52141045863017E-17,0.75,-1.22833954473516));
#17320=CARTESIAN_POINT('',(-0.143317017690053,0.75,-1.23958209161204));
#17321=CARTESIAN_POINT('Origin',(0.,0.75,0.));
#17322=CARTESIAN_POINT('',(-0.246749348660852,0.75,-1.22320001975977));
#17323=CARTESIAN_POINT('Origin',(-0.192154639568406,0.75,-1.21321664662686));
#17324=CARTESIAN_POINT('',(-0.335465908756113,0.75,-1.20190105810224));
#17325=CARTESIAN_POINT('Origin',(0.,0.75,0.));
#17326=CARTESIAN_POINT('',(-0.435062095450087,0.75,-1.16954029537568));
#17327=CARTESIAN_POINT('Origin',(-0.379577794185951,0.75,-1.1682203282434));
#17328=CARTESIAN_POINT('',(-0.519354515801077,0.75,-1.13462523166105));
#17329=CARTESIAN_POINT('Origin',(0.,0.75,0.));
#17330=CARTESIAN_POINT('',(-0.612662169561028,0.75,-1.08708260743774));
#17331=CARTESIAN_POINT('Origin',(-0.557654483764164,0.75,-1.0944585482776));
#17332=CARTESIAN_POINT('',(-0.690454891028201,0.75,-1.0394111664111));
#17333=CARTESIAN_POINT('Origin',(0.,0.75,0.));
#17334=CARTESIAN_POINT('',(-0.775176467748211,0.75,-0.977857337884348));
#17335=CARTESIAN_POINT('Origin',(-0.721999869202979,0.75,-0.993747566553533));
#17336=CARTESIAN_POINT('',(-0.844553975349804,0.75,-0.918603348636233));
#17337=CARTESIAN_POINT('Origin',(0.,0.75,0.));
#17338=CARTESIAN_POINT('',(-0.918603348636233,0.75,-0.844553975349804));
#17339=CARTESIAN_POINT('Origin',(-0.86856722168183,0.75,-0.86856722168183));
#17340=CARTESIAN_POINT('',(-0.977857337884349,0.75,-0.775176467748211));
#17341=CARTESIAN_POINT('Origin',(0.,0.75,0.));
#17342=CARTESIAN_POINT('',(-1.0394111664111,0.75,-0.690454891028201));
#17343=CARTESIAN_POINT('Origin',(-0.993747566553533,0.75,-0.721999869202979));
#17344=CARTESIAN_POINT('',(-1.08708260743774,0.75,-0.612662169561029));
#17345=CARTESIAN_POINT('Origin',(0.,0.75,0.));
#17346=CARTESIAN_POINT('',(-1.13462523166105,0.75,-0.519354515801077));
#17347=CARTESIAN_POINT('Origin',(-1.0944585482776,0.75,-0.557654483764164));
#17348=CARTESIAN_POINT('',(-1.16954029537568,0.75,-0.435062095450087));
#17349=CARTESIAN_POINT('Origin',(0.,0.75,0.));
#17350=CARTESIAN_POINT('',(-1.20190105810224,0.75,-0.335465908756113));
#17351=CARTESIAN_POINT('Origin',(-1.1682203282434,0.75,-0.379577794185951));
#17352=CARTESIAN_POINT('',(-1.22320001975977,0.75,-0.246749348660852));
#17353=CARTESIAN_POINT('Origin',(0.,0.75,0.));
#17354=CARTESIAN_POINT('',(-1.23958209161204,0.75,-0.143317017690053));
#17355=CARTESIAN_POINT('Origin',(-1.21321664662686,0.75,-0.192154639568406));
#17356=CARTESIAN_POINT('',(-1.24674050008925,0.75,-0.0523608139934482));
#17357=CARTESIAN_POINT('Origin',(0.,0.75,0.));
#17358=CARTESIAN_POINT('',(-1.24674050008925,0.75,0.0523608139934479));
#17359=CARTESIAN_POINT('Origin',(-1.22833954473516,0.75,-1.50428209172603E-16));
#17360=CARTESIAN_POINT('',(-1.23958209161204,0.75,0.143317017690053));
#17361=CARTESIAN_POINT('Origin',(0.,0.75,0.));
#17362=CARTESIAN_POINT('',(-1.22320001975977,0.75,0.246749348660851));
#17363=CARTESIAN_POINT('Origin',(-1.21321664662686,0.75,0.192154639568406));
#17364=CARTESIAN_POINT('',(-1.20190105810224,0.75,0.335465908756113));
#17365=CARTESIAN_POINT('Origin',(0.,0.75,0.));
#17366=CARTESIAN_POINT('',(-1.16954029537568,0.75,0.435062095450087));
#17367=CARTESIAN_POINT('Origin',(-1.1682203282434,0.75,0.379577794185951));
#17368=CARTESIAN_POINT('',(-1.13462523166105,0.75,0.519354515801077));
#17369=CARTESIAN_POINT('Origin',(0.,0.75,0.));
#17370=CARTESIAN_POINT('',(-1.08708260743774,0.75,0.612662169561028));
#17371=CARTESIAN_POINT('Origin',(-1.0944585482776,0.75,0.557654483764164));
#17372=CARTESIAN_POINT('',(-1.0394111664111,0.75,0.690454891028201));
#17373=CARTESIAN_POINT('Origin',(0.,0.75,0.));
#17374=CARTESIAN_POINT('',(-0.977857337884348,0.75,0.775176467748211));
#17375=CARTESIAN_POINT('Origin',(-0.993747566553533,0.75,0.721999869202979));
#17376=CARTESIAN_POINT('',(-0.918603348636233,0.75,0.844553975349804));
#17377=CARTESIAN_POINT('Origin',(0.,0.75,0.));
#17378=CARTESIAN_POINT('',(-0.844553975349804,0.75,0.918603348636233));
#17379=CARTESIAN_POINT('Origin',(-0.86856722168183,0.75,0.86856722168183));
#17380=CARTESIAN_POINT('',(-0.775176467748211,0.75,0.977857337884349));
#17381=CARTESIAN_POINT('Origin',(0.,0.75,0.));
#17382=CARTESIAN_POINT('',(-0.690454891028201,0.75,1.0394111664111));
#17383=CARTESIAN_POINT('Origin',(-0.721999869202979,0.75,0.993747566553533));
#17384=CARTESIAN_POINT('',(-0.612662169561029,0.75,1.08708260743774));
#17385=CARTESIAN_POINT('Origin',(0.,0.75,0.));
#17386=CARTESIAN_POINT('',(-0.519354515801077,0.75,1.13462523166105));
#17387=CARTESIAN_POINT('Origin',(-0.557654483764164,0.75,1.0944585482776));
#17388=CARTESIAN_POINT('',(-0.435062095450087,0.75,1.16954029537568));
#17389=CARTESIAN_POINT('Origin',(0.,0.75,0.));
#17390=CARTESIAN_POINT('',(-0.335465908756113,0.75,1.20190105810224));
#17391=CARTESIAN_POINT('Origin',(-0.379577794185951,0.75,1.1682203282434));
#17392=CARTESIAN_POINT('',(-0.246749348660852,0.75,1.22320001975977));
#17393=CARTESIAN_POINT('Origin',(0.,0.75,0.));
#17394=CARTESIAN_POINT('',(-0.143317017690053,0.75,1.23958209161204));
#17395=CARTESIAN_POINT('Origin',(-0.192154639568406,0.75,1.21321664662686));
#17396=CARTESIAN_POINT('',(-0.0523608139934483,0.75,1.24674050008925));
#17397=CARTESIAN_POINT('Origin',(0.,0.75,0.));
#17398=CARTESIAN_POINT('',(0.0523608139934478,0.75,1.24674050008925));
#17399=CARTESIAN_POINT('Origin',(-2.25642313758905E-16,0.75,1.22833954473516));
#17400=CARTESIAN_POINT('',(0.143317017690053,0.75,1.23958209161204));
#17401=CARTESIAN_POINT('Origin',(0.,0.75,0.));
#17402=CARTESIAN_POINT('',(0.246749348660851,0.75,1.22320001975977));
#17403=CARTESIAN_POINT('Origin',(0.192154639568406,0.75,1.21321664662686));
#17404=CARTESIAN_POINT('',(0.335465908756113,0.75,1.20190105810224));
#17405=CARTESIAN_POINT('Origin',(0.,0.75,0.));
#17406=CARTESIAN_POINT('',(0.435062095450087,0.75,1.16954029537568));
#17407=CARTESIAN_POINT('Origin',(0.379577794185951,0.75,1.1682203282434));
#17408=CARTESIAN_POINT('',(0.519354515801077,0.75,1.13462523166105));
#17409=CARTESIAN_POINT('Origin',(0.,0.75,0.));
#17410=CARTESIAN_POINT('',(0.612662169561028,0.75,1.08708260743774));
#17411=CARTESIAN_POINT('Origin',(0.557654483764164,0.75,1.0944585482776));
#17412=CARTESIAN_POINT('',(0.690454891028201,0.75,1.0394111664111));
#17413=CARTESIAN_POINT('Origin',(0.,0.75,0.));
#17414=CARTESIAN_POINT('',(0.775176467748211,0.75,0.977857337884349));
#17415=CARTESIAN_POINT('Origin',(0.721999869202979,0.75,0.993747566553533));
#17416=CARTESIAN_POINT('',(0.844553975349804,0.75,0.918603348636233));
#17417=CARTESIAN_POINT('Origin',(0.,0.75,0.));
#17418=CARTESIAN_POINT('',(0.918603348636233,0.75,0.844553975349804));
#17419=CARTESIAN_POINT('Origin',(0.86856722168183,0.75,0.86856722168183));
#17420=CARTESIAN_POINT('',(0.977857337884349,0.75,0.775176467748211));
#17421=CARTESIAN_POINT('Origin',(0.,0.75,0.));
#17422=CARTESIAN_POINT('',(1.0394111664111,0.75,0.690454891028201));
#17423=CARTESIAN_POINT('Origin',(0.993747566553533,0.75,0.72199986920298));
#17424=CARTESIAN_POINT('',(1.08708260743774,0.75,0.612662169561029));
#17425=CARTESIAN_POINT('Origin',(0.,0.75,0.));
#17426=CARTESIAN_POINT('',(1.13462523166105,0.75,0.519354515801077));
#17427=CARTESIAN_POINT('Origin',(1.0944585482776,0.75,0.557654483764164));
#17428=CARTESIAN_POINT('',(1.16954029537568,0.75,0.435062095450087));
#17429=CARTESIAN_POINT('Origin',(0.,0.75,0.));
#17430=CARTESIAN_POINT('',(1.20190105810224,0.75,0.335465908756113));
#17431=CARTESIAN_POINT('Origin',(1.1682203282434,0.75,0.379577794185952));
#17432=CARTESIAN_POINT('Origin',(0.,0.75,0.));
#17433=CARTESIAN_POINT('Origin',(0.,0.75,0.));
#17434=CARTESIAN_POINT('',(-1.4,0.85,1.71450551880629E-16));
#17435=CARTESIAN_POINT('Origin',(0.,0.85,0.));
#17436=CARTESIAN_POINT('',(-1.4,0.75,1.71450551880629E-16));
#17437=CARTESIAN_POINT('Origin',(0.,0.85,0.));
#17438=CARTESIAN_POINT('Origin',(1.21321664662686,0.,0.192154639568406));
#17439=CARTESIAN_POINT('',(1.23958209161204,0.,0.14331701769005));
#17440=CARTESIAN_POINT('',(1.22320001975977,0.,0.246749348660855));
#17441=CARTESIAN_POINT('Origin',(0.,0.,0.));
#17442=CARTESIAN_POINT('',(1.20190105810224,0.,0.33546590875611));
#17443=CARTESIAN_POINT('Origin',(1.1682203282434,0.,0.379577794185952));
#17444=CARTESIAN_POINT('',(1.16954029537568,0.,0.43506209545009));
#17445=CARTESIAN_POINT('Origin',(0.,0.,0.));
#17446=CARTESIAN_POINT('',(1.13462523166105,0.,0.519354515801074));
#17447=CARTESIAN_POINT('Origin',(1.0944585482776,0.,0.557654483764164));
#17448=CARTESIAN_POINT('',(1.08708260743774,0.,0.612662169561031));
#17449=CARTESIAN_POINT('Origin',(0.,0.,0.));
#17450=CARTESIAN_POINT('',(1.03941116641111,0.,0.690454891028199));
#17451=CARTESIAN_POINT('Origin',(0.993747566553533,0.,0.72199986920298));
#17452=CARTESIAN_POINT('',(0.977857337884347,0.,0.775176467748214));
#17453=CARTESIAN_POINT('Origin',(0.,0.,0.));
#17454=CARTESIAN_POINT('',(0.918603348636235,0.,0.844553975349802));
#17455=CARTESIAN_POINT('Origin',(0.86856722168183,0.,0.86856722168183));
#17456=CARTESIAN_POINT('',(0.844553975349802,0.,0.918603348636235));
#17457=CARTESIAN_POINT('Origin',(0.,0.,0.));
#17458=CARTESIAN_POINT('',(0.775176467748213,0.,0.977857337884347));
#17459=CARTESIAN_POINT('Origin',(0.721999869202979,0.,0.993747566553533));
#17460=CARTESIAN_POINT('',(0.690454891028198,0.,1.03941116641111));
#17461=CARTESIAN_POINT('Origin',(0.,0.,0.));
#17462=CARTESIAN_POINT('',(0.612662169561031,0.,1.08708260743774));
#17463=CARTESIAN_POINT('Origin',(0.557654483764164,0.,1.0944585482776));
#17464=CARTESIAN_POINT('',(0.519354515801074,0.,1.13462523166105));
#17465=CARTESIAN_POINT('Origin',(0.,0.,0.));
#17466=CARTESIAN_POINT('',(0.43506209545009,0.,1.16954029537568));
#17467=CARTESIAN_POINT('Origin',(0.379577794185951,0.,1.1682203282434));
#17468=CARTESIAN_POINT('',(0.33546590875611,0.,1.20190105810224));
#17469=CARTESIAN_POINT('Origin',(0.,0.,0.));
#17470=CARTESIAN_POINT('',(0.246749348660854,0.,1.22320001975977));
#17471=CARTESIAN_POINT('Origin',(0.192154639568406,0.,1.21321664662686));
#17472=CARTESIAN_POINT('',(0.14331701769005,0.,1.23958209161204));
#17473=CARTESIAN_POINT('Origin',(0.,0.,0.));
#17474=CARTESIAN_POINT('',(0.0523608139934508,0.,1.24674050008925));
#17475=CARTESIAN_POINT('Origin',(-2.25642313758905E-16,0.,1.22833954473516));
#17476=CARTESIAN_POINT('',(-0.0523608139934513,0.,1.24674050008925));
#17477=CARTESIAN_POINT('Origin',(0.,0.,0.));
#17478=CARTESIAN_POINT('',(-0.14331701769005,0.,1.23958209161204));
#17479=CARTESIAN_POINT('Origin',(-0.192154639568406,0.,1.21321664662686));
#17480=CARTESIAN_POINT('',(-0.246749348660855,0.,1.22320001975977));
#17481=CARTESIAN_POINT('Origin',(0.,0.,0.));
#17482=CARTESIAN_POINT('',(-0.33546590875611,0.,1.20190105810224));
#17483=CARTESIAN_POINT('Origin',(-0.379577794185951,0.,1.1682203282434));
#17484=CARTESIAN_POINT('',(-0.43506209545009,0.,1.16954029537568));
#17485=CARTESIAN_POINT('Origin',(0.,0.,0.));
#17486=CARTESIAN_POINT('',(-0.519354515801074,0.,1.13462523166105));
#17487=CARTESIAN_POINT('Origin',(-0.557654483764164,0.,1.0944585482776));
#17488=CARTESIAN_POINT('',(-0.612662169561031,0.,1.08708260743774));
#17489=CARTESIAN_POINT('Origin',(0.,0.,0.));
#17490=CARTESIAN_POINT('',(-0.690454891028199,0.,1.03941116641111));
#17491=CARTESIAN_POINT('Origin',(-0.721999869202979,0.,0.993747566553533));
#17492=CARTESIAN_POINT('',(-0.775176467748213,0.,0.977857337884347));
#17493=CARTESIAN_POINT('Origin',(0.,0.,0.));
#17494=CARTESIAN_POINT('',(-0.844553975349802,0.,0.918603348636235));
#17495=CARTESIAN_POINT('Origin',(-0.86856722168183,0.,0.86856722168183));
#17496=CARTESIAN_POINT('',(-0.918603348636235,0.,0.844553975349802));
#17497=CARTESIAN_POINT('Origin',(0.,0.,0.));
#17498=CARTESIAN_POINT('',(-0.977857337884347,0.,0.775176467748213));
#17499=CARTESIAN_POINT('Origin',(-0.993747566553533,0.,0.721999869202979));
#17500=CARTESIAN_POINT('',(-1.03941116641111,0.,0.690454891028198));
#17501=CARTESIAN_POINT('Origin',(0.,0.,0.));
#17502=CARTESIAN_POINT('',(-1.08708260743774,0.,0.612662169561031));
#17503=CARTESIAN_POINT('Origin',(-1.0944585482776,0.,0.557654483764164));
#17504=CARTESIAN_POINT('',(-1.13462523166105,0.,0.519354515801074));
#17505=CARTESIAN_POINT('Origin',(0.,0.,0.));
#17506=CARTESIAN_POINT('',(-1.16954029537568,0.,0.43506209545009));
#17507=CARTESIAN_POINT('Origin',(-1.1682203282434,0.,0.379577794185951));
#17508=CARTESIAN_POINT('',(-1.20190105810224,0.,0.33546590875611));
#17509=CARTESIAN_POINT('Origin',(0.,0.,0.));
#17510=CARTESIAN_POINT('',(-1.22320001975977,0.,0.246749348660854));
#17511=CARTESIAN_POINT('Origin',(-1.21321664662686,0.,0.192154639568406));
#17512=CARTESIAN_POINT('',(-1.23958209161204,0.,0.14331701769005));
#17513=CARTESIAN_POINT('Origin',(0.,0.,0.));
#17514=CARTESIAN_POINT('',(-1.24674050008925,0.,0.0523608139934509));
#17515=CARTESIAN_POINT('Origin',(-1.22833954473516,0.,-1.50428209172603E-16));
#17516=CARTESIAN_POINT('',(-1.24674050008925,0.,-0.0523608139934512));
#17517=CARTESIAN_POINT('Origin',(0.,0.,0.));
#17518=CARTESIAN_POINT('',(-1.23958209161204,0.,-0.14331701769005));
#17519=CARTESIAN_POINT('Origin',(-1.21321664662686,0.,-0.192154639568406));
#17520=CARTESIAN_POINT('',(-1.22320001975977,0.,-0.246749348660855));
#17521=CARTESIAN_POINT('Origin',(0.,0.,0.));
#17522=CARTESIAN_POINT('',(-1.20190105810224,0.,-0.33546590875611));
#17523=CARTESIAN_POINT('Origin',(-1.1682203282434,0.,-0.379577794185951));
#17524=CARTESIAN_POINT('',(-1.16954029537568,0.,-0.43506209545009));
#17525=CARTESIAN_POINT('Origin',(0.,0.,0.));
#17526=CARTESIAN_POINT('',(-1.13462523166105,0.,-0.519354515801074));
#17527=CARTESIAN_POINT('Origin',(-1.0944585482776,0.,-0.557654483764164));
#17528=CARTESIAN_POINT('',(-1.08708260743774,0.,-0.612662169561031));
#17529=CARTESIAN_POINT('Origin',(0.,0.,0.));
#17530=CARTESIAN_POINT('',(-1.03941116641111,0.,-0.690454891028199));
#17531=CARTESIAN_POINT('Origin',(-0.993747566553533,0.,-0.721999869202979));
#17532=CARTESIAN_POINT('',(-0.977857337884347,0.,-0.775176467748213));
#17533=CARTESIAN_POINT('Origin',(0.,0.,0.));
#17534=CARTESIAN_POINT('',(-0.918603348636235,0.,-0.844553975349802));
#17535=CARTESIAN_POINT('Origin',(-0.86856722168183,0.,-0.86856722168183));
#17536=CARTESIAN_POINT('',(-0.844553975349802,0.,-0.918603348636235));
#17537=CARTESIAN_POINT('Origin',(0.,0.,0.));
#17538=CARTESIAN_POINT('',(-0.775176467748213,0.,-0.977857337884347));
#17539=CARTESIAN_POINT('Origin',(-0.721999869202979,0.,-0.993747566553533));
#17540=CARTESIAN_POINT('',(-0.690454891028198,0.,-1.03941116641111));
#17541=CARTESIAN_POINT('Origin',(0.,0.,0.));
#17542=CARTESIAN_POINT('',(-0.612662169561031,0.,-1.08708260743774));
#17543=CARTESIAN_POINT('Origin',(-0.557654483764164,0.,-1.0944585482776));
#17544=CARTESIAN_POINT('',(-0.519354515801074,0.,-1.13462523166105));
#17545=CARTESIAN_POINT('Origin',(0.,0.,0.));
#17546=CARTESIAN_POINT('',(-0.43506209545009,0.,-1.16954029537568));
#17547=CARTESIAN_POINT('Origin',(-0.379577794185951,0.,-1.1682203282434));
#17548=CARTESIAN_POINT('',(-0.33546590875611,0.,-1.20190105810224));
#17549=CARTESIAN_POINT('Origin',(0.,0.,0.));
#17550=CARTESIAN_POINT('',(-0.246749348660854,0.,-1.22320001975977));
#17551=CARTESIAN_POINT('Origin',(-0.192154639568406,0.,-1.21321664662686));
#17552=CARTESIAN_POINT('',(-0.14331701769005,0.,-1.23958209161204));
#17553=CARTESIAN_POINT('Origin',(0.,0.,0.));
#17554=CARTESIAN_POINT('',(-0.052360813993451,0.,-1.24674050008925));
#17555=CARTESIAN_POINT('Origin',(7.52141045863017E-17,0.,-1.22833954473516));
#17556=CARTESIAN_POINT('',(0.0523608139934511,0.,-1.24674050008925));
#17557=CARTESIAN_POINT('Origin',(0.,0.,0.));
#17558=CARTESIAN_POINT('',(0.14331701769005,0.,-1.23958209161204));
#17559=CARTESIAN_POINT('Origin',(0.192154639568406,0.,-1.21321664662686));
#17560=CARTESIAN_POINT('',(0.246749348660855,0.,-1.22320001975977));
#17561=CARTESIAN_POINT('Origin',(0.,0.,0.));
#17562=CARTESIAN_POINT('',(0.33546590875611,0.,-1.20190105810224));
#17563=CARTESIAN_POINT('Origin',(0.379577794185951,0.,-1.1682203282434));
#17564=CARTESIAN_POINT('',(0.43506209545009,0.,-1.16954029537568));
#17565=CARTESIAN_POINT('Origin',(0.,0.,0.));
#17566=CARTESIAN_POINT('',(0.519354515801074,0.,-1.13462523166105));
#17567=CARTESIAN_POINT('Origin',(0.557654483764164,0.,-1.0944585482776));
#17568=CARTESIAN_POINT('',(0.612662169561031,0.,-1.08708260743774));
#17569=CARTESIAN_POINT('Origin',(0.,0.,0.));
#17570=CARTESIAN_POINT('',(0.690454891028198,0.,-1.03941116641111));
#17571=CARTESIAN_POINT('Origin',(0.721999869202979,0.,-0.993747566553533));
#17572=CARTESIAN_POINT('',(0.775176467748213,0.,-0.977857337884347));
#17573=CARTESIAN_POINT('Origin',(0.,0.,0.));
#17574=CARTESIAN_POINT('',(0.844553975349802,0.,-0.918603348636235));
#17575=CARTESIAN_POINT('Origin',(0.86856722168183,0.,-0.86856722168183));
#17576=CARTESIAN_POINT('',(0.918603348636235,0.,-0.844553975349802));
#17577=CARTESIAN_POINT('Origin',(0.,0.,0.));
#17578=CARTESIAN_POINT('',(0.977857337884347,0.,-0.775176467748213));
#17579=CARTESIAN_POINT('Origin',(0.993747566553533,0.,-0.721999869202979));
#17580=CARTESIAN_POINT('',(1.03941116641111,0.,-0.690454891028198));
#17581=CARTESIAN_POINT('Origin',(0.,0.,0.));
#17582=CARTESIAN_POINT('',(1.08708260743774,0.,-0.612662169561031));
#17583=CARTESIAN_POINT('Origin',(1.0944585482776,0.,-0.557654483764164));
#17584=CARTESIAN_POINT('',(1.13462523166105,0.,-0.519354515801074));
#17585=CARTESIAN_POINT('Origin',(0.,0.,0.));
#17586=CARTESIAN_POINT('',(1.16954029537568,0.,-0.43506209545009));
#17587=CARTESIAN_POINT('Origin',(1.1682203282434,0.,-0.379577794185951));
#17588=CARTESIAN_POINT('',(1.20190105810224,0.,-0.33546590875611));
#17589=CARTESIAN_POINT('Origin',(0.,0.,0.));
#17590=CARTESIAN_POINT('',(1.22320001975977,0.,-0.246749348660855));
#17591=CARTESIAN_POINT('Origin',(1.21321664662686,0.,-0.192154639568406));
#17592=CARTESIAN_POINT('',(1.23958209161204,0.,-0.14331701769005));
#17593=CARTESIAN_POINT('Origin',(0.,0.,0.));
#17594=CARTESIAN_POINT('',(1.24674050008925,0.,0.052360813993451));
#17595=CARTESIAN_POINT('Origin',(1.22833954473516,0.,0.));
#17596=CARTESIAN_POINT('',(1.24674050008925,0.,-0.052360813993451));
#17597=CARTESIAN_POINT('Origin',(0.,0.,0.));
#17778=UNCERTAINTY_MEASURE_WITH_UNIT(LENGTH_MEASURE(0.001),#17831,
'DISTANCE_ACCURACY_VALUE',
'Maximum model space distance between geometric entities at asserted c
onnectivities');
#17780=UNCERTAINTY_MEASURE_WITH_UNIT(LENGTH_MEASURE(0.001),#17831,
'DISTANCE_ACCURACY_VALUE',
'Maximum model space distance between geometric entities at asserted c
onnectivities');
#17828=(
GEOMETRIC_REPRESENTATION_CONTEXT(3)
GLOBAL_UNCERTAINTY_ASSIGNED_CONTEXT((#17778))
GLOBAL_UNIT_ASSIGNED_CONTEXT((#17831,#17833,#17834))
REPRESENTATION_CONTEXT('','3D')
);
#17830=(
GEOMETRIC_REPRESENTATION_CONTEXT(3)
GLOBAL_UNCERTAINTY_ASSIGNED_CONTEXT((#17780))
GLOBAL_UNIT_ASSIGNED_CONTEXT((#17831,#17833,#17834))
REPRESENTATION_CONTEXT('','3D')
);
#17831=(
LENGTH_UNIT()
NAMED_UNIT(*)
SI_UNIT(.CENTI.,.METRE.)
);
#17833=(
NAMED_UNIT(*)
PLANE_ANGLE_UNIT()
SI_UNIT($,.RADIAN.)
);
#17834=(
NAMED_UNIT(*)
SI_UNIT($,.STERADIAN.)
SOLID_ANGLE_UNIT()
);
#17882=SHAPE_DEFINITION_REPRESENTATION(#17941,#18053);
#17941=PRODUCT_DEFINITION_SHAPE('',$,#18103);
#18053=SHAPE_REPRESENTATION('',(#10458),#17828);
#18055=PRODUCT_DEFINITION_CONTEXT('part definition',#18204,'design');
#18103=PRODUCT_DEFINITION(
'Timing Pulley - 2 mm Pitch, 40 Teeth, 12 mm Bore',
'Timing Pulley - 2 mm Pitch, 40 Teeth, 12 mm Bore',#18152,#18055);
#18152=PRODUCT_DEFINITION_FORMATION('',$,#18253);
#18204=APPLICATION_CONTEXT(
'Core Data for Automotive Mechanical Design Process');
#18205=PRODUCT_CONTEXT('part definition',#18204,'mechanical');
#18253=PRODUCT('Timing Pulley - 2 mm Pitch, 40 Teeth, 12 mm Bore',
'Timing Pulley - 2 mm Pitch, 40 Teeth, 12 mm Bore',
'Timing Pulley - 2 mm Pitch, 40 Teeth, 12 mm Bore',(#18205));
#18304=COLOUR_RGB('Sky Blue',0.24,0.69,0.87);
#18305=FILL_AREA_STYLE_COLOUR('',#18304);
#18306=FILL_AREA_STYLE('',(#18305));
#18307=SURFACE_STYLE_FILL_AREA(#18306);
#18308=SURFACE_SIDE_STYLE('',(#18307));
#18309=SURFACE_STYLE_USAGE(.BOTH.,#18308);
#18310=PRESENTATION_STYLE_ASSIGNMENT((#18309));
ENDSEC;
END-ISO-10303-21;
